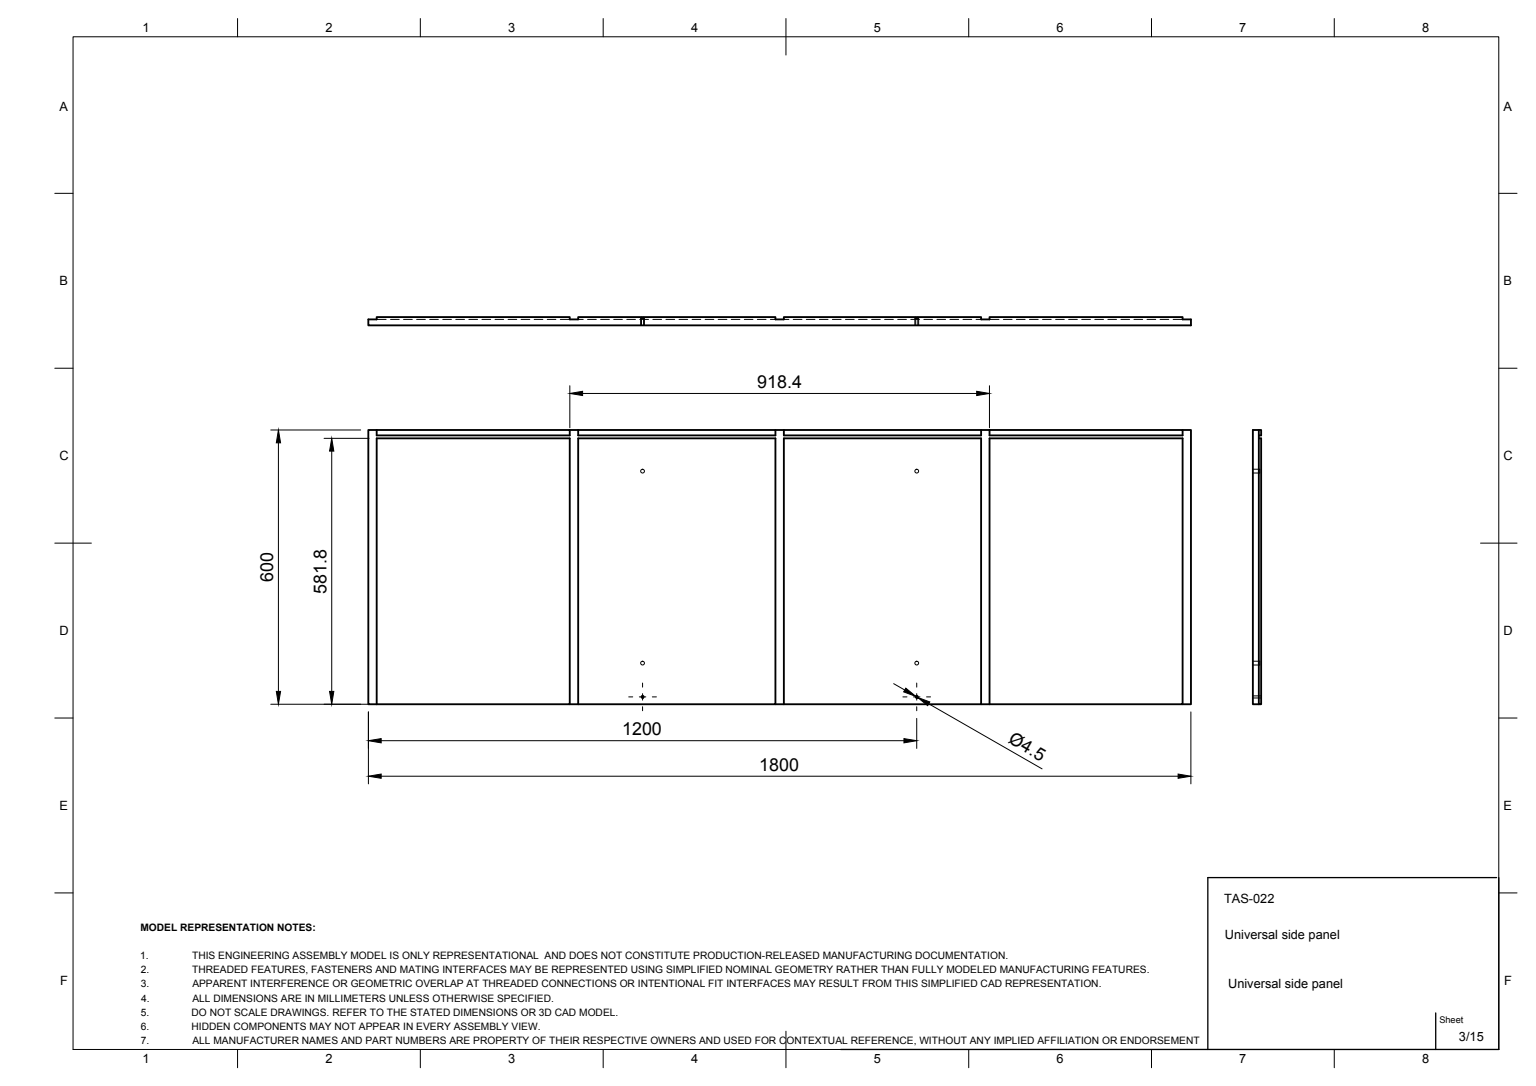
ISO-10303-21;
HEADER;
/* Generated by software containing ST-Developer
 * from STEP Tools, Inc. (www.steptools.com) 
 */

FILE_DESCRIPTION(
/* description */ (''),
/* implementation_level */ '2;1');

FILE_NAME(
/* name */ 'Universal side panel.step',
/* time_stamp */ '2026-11-15T21:02:08-08:00',
/* author */ (''),
/* organization */ (''),
/* preprocessor_version */ 'ST-DEVELOPER v20.2',
/* originating_system */ 'Autodesk Translation Framework v15.17.0.0',
/* authorisation */ '');

FILE_SCHEMA (('AUTOMOTIVE_DESIGN { 1 0 10303 214 3 1 1 }'));
ENDSEC;

DATA;
#10=MECHANICAL_DESIGN_GEOMETRIC_PRESENTATION_REPRESENTATION('',(#608),#31566);
#401=FACE_BOUND('',#1014,.T.);
#402=FACE_BOUND('',#1021,.T.);
#403=FACE_BOUND('',#1035,.T.);
#404=FACE_BOUND('',#1036,.T.);
#405=FACE_BOUND('',#1037,.T.);
#406=FACE_BOUND('',#1038,.T.);
#407=FACE_BOUND('',#1039,.T.);
#408=FACE_BOUND('',#1040,.T.);
#457=CIRCLE('',#6010,0.409999999999997);
#458=CIRCLE('',#6011,0.409999999999997);
#459=CIRCLE('',#6014,0.409999999999997);
#460=CIRCLE('',#6015,0.409999999999997);
#461=CIRCLE('',#6018,0.409999999999997);
#462=CIRCLE('',#6019,0.409999999999997);
#463=CIRCLE('',#6022,0.409999999999997);
#464=CIRCLE('',#6023,0.409999999999997);
#465=CIRCLE('',#6026,0.225000000000001);
#466=CIRCLE('',#6027,0.225000000000001);
#467=CIRCLE('',#6029,0.224999999999994);
#468=CIRCLE('',#6030,0.224999999999994);
#510=CYLINDRICAL_SURFACE('',#6009,0.409999999999997);
#511=CYLINDRICAL_SURFACE('',#6013,0.409999999999997);
#512=CYLINDRICAL_SURFACE('',#6017,0.409999999999997);
#513=CYLINDRICAL_SURFACE('',#6021,0.409999999999997);
#514=CYLINDRICAL_SURFACE('',#6025,0.225000000000001);
#515=CYLINDRICAL_SURFACE('',#6028,0.224999999999994);
#578=SHAPE_REPRESENTATION_RELATIONSHIP('SRR','None',#31642,#593);
#593=ADVANCED_BREP_SHAPE_REPRESENTATION('',(#623),#31557);
#608=STYLED_ITEM('',(#31723),#623);
#623=MANIFOLD_SOLID_BREP('Body1',#5721);
#697=FACE_OUTER_BOUND('',#986,.T.);
#698=FACE_OUTER_BOUND('',#987,.T.);
#699=FACE_OUTER_BOUND('',#988,.T.);
#700=FACE_OUTER_BOUND('',#989,.T.);
#701=FACE_OUTER_BOUND('',#990,.T.);
#702=FACE_OUTER_BOUND('',#991,.T.);
#703=FACE_OUTER_BOUND('',#992,.T.);
#704=FACE_OUTER_BOUND('',#993,.T.);
#705=FACE_OUTER_BOUND('',#994,.T.);
#706=FACE_OUTER_BOUND('',#995,.T.);
#707=FACE_OUTER_BOUND('',#996,.T.);
#708=FACE_OUTER_BOUND('',#997,.T.);
#709=FACE_OUTER_BOUND('',#998,.T.);
#710=FACE_OUTER_BOUND('',#999,.T.);
#711=FACE_OUTER_BOUND('',#1000,.T.);
#712=FACE_OUTER_BOUND('',#1001,.T.);
#713=FACE_OUTER_BOUND('',#1002,.T.);
#714=FACE_OUTER_BOUND('',#1003,.T.);
#715=FACE_OUTER_BOUND('',#1004,.T.);
#716=FACE_OUTER_BOUND('',#1005,.T.);
#717=FACE_OUTER_BOUND('',#1006,.T.);
#718=FACE_OUTER_BOUND('',#1007,.T.);
#719=FACE_OUTER_BOUND('',#1008,.T.);
#720=FACE_OUTER_BOUND('',#1009,.T.);
#721=FACE_OUTER_BOUND('',#1010,.T.);
#722=FACE_OUTER_BOUND('',#1011,.T.);
#723=FACE_OUTER_BOUND('',#1012,.T.);
#724=FACE_OUTER_BOUND('',#1013,.T.);
#725=FACE_OUTER_BOUND('',#1015,.T.);
#726=FACE_OUTER_BOUND('',#1016,.T.);
#727=FACE_OUTER_BOUND('',#1017,.T.);
#728=FACE_OUTER_BOUND('',#1018,.T.);
#729=FACE_OUTER_BOUND('',#1019,.T.);
#730=FACE_OUTER_BOUND('',#1020,.T.);
#731=FACE_OUTER_BOUND('',#1022,.T.);
#732=FACE_OUTER_BOUND('',#1023,.T.);
#733=FACE_OUTER_BOUND('',#1024,.T.);
#734=FACE_OUTER_BOUND('',#1025,.T.);
#735=FACE_OUTER_BOUND('',#1026,.T.);
#736=FACE_OUTER_BOUND('',#1027,.T.);
#737=FACE_OUTER_BOUND('',#1028,.T.);
#738=FACE_OUTER_BOUND('',#1029,.T.);
#739=FACE_OUTER_BOUND('',#1030,.T.);
#740=FACE_OUTER_BOUND('',#1031,.T.);
#741=FACE_OUTER_BOUND('',#1032,.T.);
#742=FACE_OUTER_BOUND('',#1033,.T.);
#743=FACE_OUTER_BOUND('',#1034,.T.);
#744=FACE_OUTER_BOUND('',#1041,.T.);
#986=EDGE_LOOP('',(#3945,#3946,#3947,#3948));
#987=EDGE_LOOP('',(#3949));
#988=EDGE_LOOP('',(#3950,#3951,#3952,#3953));
#989=EDGE_LOOP('',(#3954));
#990=EDGE_LOOP('',(#3955,#3956,#3957,#3958));
#991=EDGE_LOOP('',(#3959));
#992=EDGE_LOOP('',(#3960,#3961,#3962,#3963));
#993=EDGE_LOOP('',(#3964));
#994=EDGE_LOOP('',(#3965,#3966,#3967,#3968));
#995=EDGE_LOOP('',(#3969,#3970,#3971,#3972));
#996=EDGE_LOOP('',(#3973,#3974,#3975,#3976));
#997=EDGE_LOOP('',(#3977,#3978,#3979,#3980));
#998=EDGE_LOOP('',(#3981,#3982,#3983,#3984));
#999=EDGE_LOOP('',(#3985,#3986,#3987,#3988));
#1000=EDGE_LOOP('',(#3989,#3990,#3991,#3992));
#1001=EDGE_LOOP('',(#3993,#3994,#3995,#3996));
#1002=EDGE_LOOP('',(#3997,#3998,#3999,#4000));
#1003=EDGE_LOOP('',(#4001,#4002,#4003,#4004));
#1004=EDGE_LOOP('',(#4005,#4006,#4007,#4008,#4009,#4010,#4011,#4012,#4013,
#4014,#4015,#4016,#4017,#4018,#4019,#4020,#4021,#4022,#4023,#4024,#4025,
#4026,#4027,#4028,#4029,#4030,#4031,#4032,#4033,#4034,#4035,#4036,#4037,
#4038,#4039,#4040));
#1005=EDGE_LOOP('',(#4041,#4042,#4043,#4044));
#1006=EDGE_LOOP('',(#4045,#4046,#4047,#4048));
#1007=EDGE_LOOP('',(#4049,#4050,#4051,#4052));
#1008=EDGE_LOOP('',(#4053,#4054,#4055,#4056));
#1009=EDGE_LOOP('',(#4057,#4058,#4059,#4060));
#1010=EDGE_LOOP('',(#4061,#4062,#4063,#4064));
#1011=EDGE_LOOP('',(#4065,#4066,#4067,#4068));
#1012=EDGE_LOOP('',(#4069,#4070,#4071,#4072));
#1013=EDGE_LOOP('',(#4073,#4074,#4075,#4076));
#1014=EDGE_LOOP('',(#4077));
#1015=EDGE_LOOP('',(#4078,#4079,#4080,#4081));
#1016=EDGE_LOOP('',(#4082,#4083,#4084,#4085));
#1017=EDGE_LOOP('',(#4086,#4087,#4088,#4089));
#1018=EDGE_LOOP('',(#4090,#4091,#4092,#4093));
#1019=EDGE_LOOP('',(#4094,#4095,#4096,#4097));
#1020=EDGE_LOOP('',(#4098,#4099,#4100,#4101));
#1021=EDGE_LOOP('',(#4102));
#1022=EDGE_LOOP('',(#4103,#4104,#4105,#4106));
#1023=EDGE_LOOP('',(#4107,#4108,#4109,#4110));
#1024=EDGE_LOOP('',(#4111,#4112,#4113,#4114));
#1025=EDGE_LOOP('',(#4115,#4116,#4117,#4118));
#1026=EDGE_LOOP('',(#4119,#4120,#4121,#4122));
#1027=EDGE_LOOP('',(#4123,#4124,#4125,#4126));
#1028=EDGE_LOOP('',(#4127,#4128,#4129,#4130));
#1029=EDGE_LOOP('',(#4131,#4132,#4133,#4134));
#1030=EDGE_LOOP('',(#4135,#4136,#4137,#4138));
#1031=EDGE_LOOP('',(#4139,#4140,#4141,#4142,#4143,#4144,#4145,#4146,#4147,
#4148,#4149,#4150,#4151,#4152,#4153,#4154,#4155,#4156,#4157,#4158));
#1032=EDGE_LOOP('',(#4159,#4160,#4161,#4162));
#1033=EDGE_LOOP('',(#4163,#4164,#4165,#4166,#4167,#4168,#4169,#4170,#4171,
#4172,#4173,#4174,#4175,#4176,#4177,#4178,#4179,#4180,#4181,#4182));
#1034=EDGE_LOOP('',(#4183,#4184,#4185,#4186));
#1035=EDGE_LOOP('',(#4187));
#1036=EDGE_LOOP('',(#4188));
#1037=EDGE_LOOP('',(#4189));
#1038=EDGE_LOOP('',(#4190));
#1039=EDGE_LOOP('',(#4191));
#1040=EDGE_LOOP('',(#4192));
#1041=EDGE_LOOP('',(#4193,#4194,#4195,#4196));
#1325=LINE('',#7903,#1832);
#1326=LINE('',#7910,#1833);
#1327=LINE('',#7917,#1834);
#1328=LINE('',#7924,#1835);
#1329=LINE('',#7931,#1836);
#1330=LINE('',#7937,#1837);
#1331=LINE('',#7942,#1838);
#1332=LINE('',#7944,#1839);
#1333=LINE('',#7946,#1840);
#1334=LINE('',#7947,#1841);
#1335=LINE('',#7951,#1842);
#1336=LINE('',#7953,#1843);
#1337=LINE('',#7955,#1844);
#1338=LINE('',#7956,#1845);
#1339=LINE('',#7960,#1846);
#1340=LINE('',#7962,#1847);
#1341=LINE('',#7964,#1848);
#1342=LINE('',#7965,#1849);
#1343=LINE('',#7969,#1850);
#1344=LINE('',#7971,#1851);
#1345=LINE('',#7973,#1852);
#1346=LINE('',#7974,#1853);
#1347=LINE('',#7978,#1854);
#1348=LINE('',#7980,#1855);
#1349=LINE('',#7982,#1856);
#1350=LINE('',#7983,#1857);
#1351=LINE('',#7987,#1858);
#1352=LINE('',#7989,#1859);
#1353=LINE('',#7991,#1860);
#1354=LINE('',#7992,#1861);
#1355=LINE('',#7996,#1862);
#1356=LINE('',#7998,#1863);
#1357=LINE('',#8000,#1864);
#1358=LINE('',#8001,#1865);
#1359=LINE('',#8005,#1866);
#1360=LINE('',#8007,#1867);
#1361=LINE('',#8009,#1868);
#1362=LINE('',#8010,#1869);
#1363=LINE('',#8013,#1870);
#1364=LINE('',#8015,#1871);
#1365=LINE('',#8017,#1872);
#1366=LINE('',#8019,#1873);
#1367=LINE('',#8020,#1874);
#1368=LINE('',#8022,#1875);
#1369=LINE('',#8024,#1876);
#1370=LINE('',#8025,#1877);
#1371=LINE('',#8027,#1878);
#1372=LINE('',#8029,#1879);
#1373=LINE('',#8030,#1880);
#1374=LINE('',#8032,#1881);
#1375=LINE('',#8034,#1882);
#1376=LINE('',#8035,#1883);
#1377=LINE('',#8037,#1884);
#1378=LINE('',#8039,#1885);
#1379=LINE('',#8041,#1886);
#1380=LINE('',#8043,#1887);
#1381=LINE('',#8044,#1888);
#1382=LINE('',#8046,#1889);
#1383=LINE('',#8048,#1890);
#1384=LINE('',#8049,#1891);
#1385=LINE('',#8051,#1892);
#1386=LINE('',#8053,#1893);
#1387=LINE('',#8054,#1894);
#1388=LINE('',#8056,#1895);
#1389=LINE('',#8058,#1896);
#1390=LINE('',#8059,#1897);
#1391=LINE('',#8062,#1898);
#1392=LINE('',#8063,#1899);
#1393=LINE('',#8066,#1900);
#1394=LINE('',#8067,#1901);
#1395=LINE('',#8070,#1902);
#1396=LINE('',#8071,#1903);
#1397=LINE('',#8074,#1904);
#1398=LINE('',#8075,#1905);
#1399=LINE('',#8077,#1906);
#1400=LINE('',#8079,#1907);
#1401=LINE('',#8082,#1908);
#1402=LINE('',#8083,#1909);
#1403=LINE('',#8086,#1910);
#1404=LINE('',#8087,#1911);
#1405=LINE('',#8090,#1912);
#1406=LINE('',#8091,#1913);
#1407=LINE('',#8094,#1914);
#1408=LINE('',#8095,#1915);
#1409=LINE('',#8097,#1916);
#1410=LINE('',#8099,#1917);
#1411=LINE('',#8102,#1918);
#1412=LINE('',#8103,#1919);
#1413=LINE('',#8106,#1920);
#1414=LINE('',#8107,#1921);
#1415=LINE('',#8110,#1922);
#1416=LINE('',#8111,#1923);
#1417=LINE('',#8114,#1924);
#1418=LINE('',#8115,#1925);
#1419=LINE('',#8117,#1926);
#1420=LINE('',#8119,#1927);
#1421=LINE('',#8122,#1928);
#1422=LINE('',#8123,#1929);
#1423=LINE('',#8126,#1930);
#1424=LINE('',#8127,#1931);
#1425=LINE('',#8130,#1932);
#1426=LINE('',#8131,#1933);
#1427=LINE('',#8134,#1934);
#1428=LINE('',#8135,#1935);
#1429=LINE('',#8137,#1936);
#1430=LINE('',#8139,#1937);
#1431=LINE('',#8142,#1938);
#1432=LINE('',#8144,#1939);
#1433=LINE('',#8145,#1940);
#1434=LINE('',#8148,#1941);
#1435=LINE('',#8149,#1942);
#1436=LINE('',#8152,#1943);
#1437=LINE('',#8153,#1944);
#1438=LINE('',#8155,#1945);
#1832=VECTOR('',#6631,0.409999999999997);
#1833=VECTOR('',#6640,0.409999999999997);
#1834=VECTOR('',#6649,0.409999999999997);
#1835=VECTOR('',#6658,0.409999999999997);
#1836=VECTOR('',#6667,0.225000000000001);
#1837=VECTOR('',#6674,0.224999999999994);
#1838=VECTOR('',#6679,1.);
#1839=VECTOR('',#6680,1.);
#1840=VECTOR('',#6681,1.);
#1841=VECTOR('',#6682,1.);
#1842=VECTOR('',#6685,1.);
#1843=VECTOR('',#6686,1.);
#1844=VECTOR('',#6687,1.);
#1845=VECTOR('',#6688,1.);
#1846=VECTOR('',#6691,1.);
#1847=VECTOR('',#6692,1.);
#1848=VECTOR('',#6693,1.);
#1849=VECTOR('',#6694,1.);
#1850=VECTOR('',#6697,1.);
#1851=VECTOR('',#6698,1.);
#1852=VECTOR('',#6699,1.);
#1853=VECTOR('',#6700,1.);
#1854=VECTOR('',#6703,1.);
#1855=VECTOR('',#6704,1.);
#1856=VECTOR('',#6705,1.);
#1857=VECTOR('',#6706,1.);
#1858=VECTOR('',#6709,1.);
#1859=VECTOR('',#6710,1.);
#1860=VECTOR('',#6711,1.);
#1861=VECTOR('',#6712,1.);
#1862=VECTOR('',#6715,1.);
#1863=VECTOR('',#6716,1.);
#1864=VECTOR('',#6717,1.);
#1865=VECTOR('',#6718,1.);
#1866=VECTOR('',#6721,1.);
#1867=VECTOR('',#6722,1.);
#1868=VECTOR('',#6723,1.);
#1869=VECTOR('',#6724,1.);
#1870=VECTOR('',#6727,1.);
#1871=VECTOR('',#6728,1.);
#1872=VECTOR('',#6729,1.);
#1873=VECTOR('',#6730,1.);
#1874=VECTOR('',#6731,1.);
#1875=VECTOR('',#6732,1.);
#1876=VECTOR('',#6733,1.);
#1877=VECTOR('',#6734,1.);
#1878=VECTOR('',#6735,1.);
#1879=VECTOR('',#6736,1.);
#1880=VECTOR('',#6737,1.);
#1881=VECTOR('',#6738,1.);
#1882=VECTOR('',#6739,1.);
#1883=VECTOR('',#6740,1.);
#1884=VECTOR('',#6741,1.);
#1885=VECTOR('',#6742,1.);
#1886=VECTOR('',#6743,1.);
#1887=VECTOR('',#6744,1.);
#1888=VECTOR('',#6745,1.);
#1889=VECTOR('',#6746,1.);
#1890=VECTOR('',#6747,1.);
#1891=VECTOR('',#6748,1.);
#1892=VECTOR('',#6749,1.);
#1893=VECTOR('',#6750,1.);
#1894=VECTOR('',#6751,1.);
#1895=VECTOR('',#6752,1.);
#1896=VECTOR('',#6753,1.);
#1897=VECTOR('',#6754,1.);
#1898=VECTOR('',#6757,1.);
#1899=VECTOR('',#6758,1.);
#1900=VECTOR('',#6761,1.);
#1901=VECTOR('',#6762,1.);
#1902=VECTOR('',#6765,1.);
#1903=VECTOR('',#6766,1.);
#1904=VECTOR('',#6769,1.);
#1905=VECTOR('',#6770,1.);
#1906=VECTOR('',#6773,1.);
#1907=VECTOR('',#6776,1.);
#1908=VECTOR('',#6779,1.);
#1909=VECTOR('',#6780,1.);
#1910=VECTOR('',#6783,1.);
#1911=VECTOR('',#6784,1.);
#1912=VECTOR('',#6787,1.);
#1913=VECTOR('',#6788,1.);
#1914=VECTOR('',#6791,1.);
#1915=VECTOR('',#6792,1.);
#1916=VECTOR('',#6795,1.);
#1917=VECTOR('',#6798,1.);
#1918=VECTOR('',#6801,1.);
#1919=VECTOR('',#6802,1.);
#1920=VECTOR('',#6805,1.);
#1921=VECTOR('',#6806,1.);
#1922=VECTOR('',#6809,1.);
#1923=VECTOR('',#6810,1.);
#1924=VECTOR('',#6813,1.);
#1925=VECTOR('',#6814,1.);
#1926=VECTOR('',#6817,1.);
#1927=VECTOR('',#6820,1.);
#1928=VECTOR('',#6823,1.);
#1929=VECTOR('',#6824,1.);
#1930=VECTOR('',#6827,1.);
#1931=VECTOR('',#6828,1.);
#1932=VECTOR('',#6831,1.);
#1933=VECTOR('',#6832,1.);
#1934=VECTOR('',#6835,1.);
#1935=VECTOR('',#6836,1.);
#1936=VECTOR('',#6839,1.);
#1937=VECTOR('',#6842,1.);
#1938=VECTOR('',#6845,1.);
#1939=VECTOR('',#6846,1.);
#1940=VECTOR('',#6847,1.);
#1941=VECTOR('',#6850,1.);
#1942=VECTOR('',#6851,1.);
#1943=VECTOR('',#6854,1.);
#1944=VECTOR('',#6855,1.);
#1945=VECTOR('',#6858,1.);
#2326=VERTEX_POINT('',#7900);
#2327=VERTEX_POINT('',#7902);
#2328=VERTEX_POINT('',#7907);
#2329=VERTEX_POINT('',#7909);
#2330=VERTEX_POINT('',#7914);
#2331=VERTEX_POINT('',#7916);
#2332=VERTEX_POINT('',#7921);
#2333=VERTEX_POINT('',#7923);
#2334=VERTEX_POINT('',#7928);
#2335=VERTEX_POINT('',#7930);
#2336=VERTEX_POINT('',#7934);
#2337=VERTEX_POINT('',#7936);
#2338=VERTEX_POINT('',#7940);
#2339=VERTEX_POINT('',#7941);
#2340=VERTEX_POINT('',#7943);
#2341=VERTEX_POINT('',#7945);
#2342=VERTEX_POINT('',#7949);
#2343=VERTEX_POINT('',#7950);
#2344=VERTEX_POINT('',#7952);
#2345=VERTEX_POINT('',#7954);
#2346=VERTEX_POINT('',#7958);
#2347=VERTEX_POINT('',#7959);
#2348=VERTEX_POINT('',#7961);
#2349=VERTEX_POINT('',#7963);
#2350=VERTEX_POINT('',#7967);
#2351=VERTEX_POINT('',#7968);
#2352=VERTEX_POINT('',#7970);
#2353=VERTEX_POINT('',#7972);
#2354=VERTEX_POINT('',#7976);
#2355=VERTEX_POINT('',#7977);
#2356=VERTEX_POINT('',#7979);
#2357=VERTEX_POINT('',#7981);
#2358=VERTEX_POINT('',#7985);
#2359=VERTEX_POINT('',#7986);
#2360=VERTEX_POINT('',#7988);
#2361=VERTEX_POINT('',#7990);
#2362=VERTEX_POINT('',#7994);
#2363=VERTEX_POINT('',#7995);
#2364=VERTEX_POINT('',#7997);
#2365=VERTEX_POINT('',#7999);
#2366=VERTEX_POINT('',#8003);
#2367=VERTEX_POINT('',#8004);
#2368=VERTEX_POINT('',#8006);
#2369=VERTEX_POINT('',#8008);
#2370=VERTEX_POINT('',#8012);
#2371=VERTEX_POINT('',#8014);
#2372=VERTEX_POINT('',#8016);
#2373=VERTEX_POINT('',#8018);
#2374=VERTEX_POINT('',#8021);
#2375=VERTEX_POINT('',#8023);
#2376=VERTEX_POINT('',#8026);
#2377=VERTEX_POINT('',#8028);
#2378=VERTEX_POINT('',#8031);
#2379=VERTEX_POINT('',#8033);
#2380=VERTEX_POINT('',#8036);
#2381=VERTEX_POINT('',#8038);
#2382=VERTEX_POINT('',#8040);
#2383=VERTEX_POINT('',#8042);
#2384=VERTEX_POINT('',#8045);
#2385=VERTEX_POINT('',#8047);
#2386=VERTEX_POINT('',#8050);
#2387=VERTEX_POINT('',#8052);
#2388=VERTEX_POINT('',#8055);
#2389=VERTEX_POINT('',#8057);
#2390=VERTEX_POINT('',#8061);
#2391=VERTEX_POINT('',#8065);
#2392=VERTEX_POINT('',#8069);
#2393=VERTEX_POINT('',#8073);
#2394=VERTEX_POINT('',#8081);
#2395=VERTEX_POINT('',#8085);
#2396=VERTEX_POINT('',#8089);
#2397=VERTEX_POINT('',#8093);
#2398=VERTEX_POINT('',#8101);
#2399=VERTEX_POINT('',#8105);
#2400=VERTEX_POINT('',#8109);
#2401=VERTEX_POINT('',#8113);
#2402=VERTEX_POINT('',#8121);
#2403=VERTEX_POINT('',#8125);
#2404=VERTEX_POINT('',#8129);
#2405=VERTEX_POINT('',#8133);
#2406=VERTEX_POINT('',#8141);
#2407=VERTEX_POINT('',#8143);
#2408=VERTEX_POINT('',#8147);
#2409=VERTEX_POINT('',#8151);
#2968=EDGE_CURVE('',#2326,#2326,#457,.T.);
#2969=EDGE_CURVE('',#2326,#2327,#1325,.T.);
#2970=EDGE_CURVE('',#2327,#2327,#458,.T.);
#2971=EDGE_CURVE('',#2328,#2328,#459,.T.);
#2972=EDGE_CURVE('',#2328,#2329,#1326,.T.);
#2973=EDGE_CURVE('',#2329,#2329,#460,.T.);
#2974=EDGE_CURVE('',#2330,#2330,#461,.T.);
#2975=EDGE_CURVE('',#2330,#2331,#1327,.T.);
#2976=EDGE_CURVE('',#2331,#2331,#462,.T.);
#2977=EDGE_CURVE('',#2332,#2332,#463,.T.);
#2978=EDGE_CURVE('',#2332,#2333,#1328,.T.);
#2979=EDGE_CURVE('',#2333,#2333,#464,.T.);
#2980=EDGE_CURVE('',#2334,#2334,#465,.T.);
#2981=EDGE_CURVE('',#2334,#2335,#1329,.T.);
#2982=EDGE_CURVE('',#2335,#2335,#466,.T.);
#2983=EDGE_CURVE('',#2336,#2336,#467,.T.);
#2984=EDGE_CURVE('',#2336,#2337,#1330,.T.);
#2985=EDGE_CURVE('',#2337,#2337,#468,.T.);
#2986=EDGE_CURVE('',#2338,#2339,#1331,.T.);
#2987=EDGE_CURVE('',#2340,#2338,#1332,.T.);
#2988=EDGE_CURVE('',#2341,#2340,#1333,.T.);
#2989=EDGE_CURVE('',#2339,#2341,#1334,.T.);
#2990=EDGE_CURVE('',#2342,#2343,#1335,.T.);
#2991=EDGE_CURVE('',#2344,#2342,#1336,.T.);
#2992=EDGE_CURVE('',#2345,#2344,#1337,.T.);
#2993=EDGE_CURVE('',#2343,#2345,#1338,.T.);
#2994=EDGE_CURVE('',#2346,#2347,#1339,.T.);
#2995=EDGE_CURVE('',#2348,#2346,#1340,.T.);
#2996=EDGE_CURVE('',#2349,#2348,#1341,.T.);
#2997=EDGE_CURVE('',#2347,#2349,#1342,.T.);
#2998=EDGE_CURVE('',#2350,#2351,#1343,.T.);
#2999=EDGE_CURVE('',#2352,#2350,#1344,.T.);
#3000=EDGE_CURVE('',#2353,#2352,#1345,.T.);
#3001=EDGE_CURVE('',#2351,#2353,#1346,.T.);
#3002=EDGE_CURVE('',#2354,#2355,#1347,.T.);
#3003=EDGE_CURVE('',#2356,#2354,#1348,.T.);
#3004=EDGE_CURVE('',#2357,#2356,#1349,.T.);
#3005=EDGE_CURVE('',#2357,#2355,#1350,.T.);
#3006=EDGE_CURVE('',#2358,#2359,#1351,.T.);
#3007=EDGE_CURVE('',#2360,#2358,#1352,.T.);
#3008=EDGE_CURVE('',#2361,#2360,#1353,.T.);
#3009=EDGE_CURVE('',#2361,#2359,#1354,.T.);
#3010=EDGE_CURVE('',#2362,#2363,#1355,.T.);
#3011=EDGE_CURVE('',#2364,#2362,#1356,.T.);
#3012=EDGE_CURVE('',#2365,#2364,#1357,.T.);
#3013=EDGE_CURVE('',#2365,#2363,#1358,.T.);
#3014=EDGE_CURVE('',#2366,#2367,#1359,.T.);
#3015=EDGE_CURVE('',#2368,#2366,#1360,.T.);
#3016=EDGE_CURVE('',#2369,#2368,#1361,.T.);
#3017=EDGE_CURVE('',#2369,#2367,#1362,.T.);
#3018=EDGE_CURVE('',#2370,#2350,#1363,.T.);
#3019=EDGE_CURVE('',#2371,#2370,#1364,.T.);
#3020=EDGE_CURVE('',#2372,#2371,#1365,.T.);
#3021=EDGE_CURVE('',#2373,#2372,#1366,.T.);
#3022=EDGE_CURVE('',#2367,#2373,#1367,.T.);
#3023=EDGE_CURVE('',#2369,#2374,#1368,.T.);
#3024=EDGE_CURVE('',#2375,#2374,#1369,.T.);
#3025=EDGE_CURVE('',#2363,#2375,#1370,.T.);
#3026=EDGE_CURVE('',#2365,#2376,#1371,.T.);
#3027=EDGE_CURVE('',#2377,#2376,#1372,.T.);
#3028=EDGE_CURVE('',#2359,#2377,#1373,.T.);
#3029=EDGE_CURVE('',#2361,#2378,#1374,.T.);
#3030=EDGE_CURVE('',#2379,#2378,#1375,.T.);
#3031=EDGE_CURVE('',#2355,#2379,#1376,.T.);
#3032=EDGE_CURVE('',#2357,#2380,#1377,.T.);
#3033=EDGE_CURVE('',#2381,#2380,#1378,.T.);
#3034=EDGE_CURVE('',#2382,#2381,#1379,.T.);
#3035=EDGE_CURVE('',#2383,#2382,#1380,.T.);
#3036=EDGE_CURVE('',#2383,#2348,#1381,.T.);
#3037=EDGE_CURVE('',#2384,#2346,#1382,.T.);
#3038=EDGE_CURVE('',#2385,#2384,#1383,.T.);
#3039=EDGE_CURVE('',#2385,#2344,#1384,.T.);
#3040=EDGE_CURVE('',#2386,#2342,#1385,.T.);
#3041=EDGE_CURVE('',#2387,#2386,#1386,.T.);
#3042=EDGE_CURVE('',#2387,#2340,#1387,.T.);
#3043=EDGE_CURVE('',#2388,#2338,#1388,.T.);
#3044=EDGE_CURVE('',#2389,#2388,#1389,.T.);
#3045=EDGE_CURVE('',#2389,#2352,#1390,.T.);
#3046=EDGE_CURVE('',#2390,#2373,#1391,.T.);
#3047=EDGE_CURVE('',#2366,#2390,#1392,.T.);
#3048=EDGE_CURVE('',#2391,#2351,#1393,.T.);
#3049=EDGE_CURVE('',#2370,#2391,#1394,.T.);
#3050=EDGE_CURVE('',#2392,#2390,#1395,.T.);
#3051=EDGE_CURVE('',#2392,#2368,#1396,.T.);
#3052=EDGE_CURVE('',#2353,#2393,#1397,.T.);
#3053=EDGE_CURVE('',#2393,#2391,#1398,.T.);
#3054=EDGE_CURVE('',#2374,#2392,#1399,.T.);
#3055=EDGE_CURVE('',#2393,#2389,#1400,.T.);
#3056=EDGE_CURVE('',#2394,#2375,#1401,.T.);
#3057=EDGE_CURVE('',#2362,#2394,#1402,.T.);
#3058=EDGE_CURVE('',#2395,#2339,#1403,.T.);
#3059=EDGE_CURVE('',#2388,#2395,#1404,.T.);
#3060=EDGE_CURVE('',#2396,#2394,#1405,.T.);
#3061=EDGE_CURVE('',#2396,#2364,#1406,.T.);
#3062=EDGE_CURVE('',#2341,#2397,#1407,.T.);
#3063=EDGE_CURVE('',#2397,#2395,#1408,.T.);
#3064=EDGE_CURVE('',#2376,#2396,#1409,.T.);
#3065=EDGE_CURVE('',#2397,#2387,#1410,.T.);
#3066=EDGE_CURVE('',#2398,#2377,#1411,.T.);
#3067=EDGE_CURVE('',#2358,#2398,#1412,.T.);
#3068=EDGE_CURVE('',#2399,#2343,#1413,.T.);
#3069=EDGE_CURVE('',#2386,#2399,#1414,.T.);
#3070=EDGE_CURVE('',#2400,#2398,#1415,.T.);
#3071=EDGE_CURVE('',#2400,#2360,#1416,.T.);
#3072=EDGE_CURVE('',#2345,#2401,#1417,.T.);
#3073=EDGE_CURVE('',#2401,#2399,#1418,.T.);
#3074=EDGE_CURVE('',#2378,#2400,#1419,.T.);
#3075=EDGE_CURVE('',#2401,#2385,#1420,.T.);
#3076=EDGE_CURVE('',#2402,#2379,#1421,.T.);
#3077=EDGE_CURVE('',#2354,#2402,#1422,.T.);
#3078=EDGE_CURVE('',#2403,#2347,#1423,.T.);
#3079=EDGE_CURVE('',#2384,#2403,#1424,.T.);
#3080=EDGE_CURVE('',#2404,#2402,#1425,.T.);
#3081=EDGE_CURVE('',#2404,#2356,#1426,.T.);
#3082=EDGE_CURVE('',#2349,#2405,#1427,.T.);
#3083=EDGE_CURVE('',#2405,#2403,#1428,.T.);
#3084=EDGE_CURVE('',#2380,#2404,#1429,.T.);
#3085=EDGE_CURVE('',#2405,#2383,#1430,.T.);
#3086=EDGE_CURVE('',#2382,#2406,#1431,.T.);
#3087=EDGE_CURVE('',#2406,#2407,#1432,.T.);
#3088=EDGE_CURVE('',#2371,#2407,#1433,.T.);
#3089=EDGE_CURVE('',#2408,#2381,#1434,.T.);
#3090=EDGE_CURVE('',#2406,#2408,#1435,.T.);
#3091=EDGE_CURVE('',#2409,#2372,#1436,.T.);
#3092=EDGE_CURVE('',#2408,#2409,#1437,.T.);
#3093=EDGE_CURVE('',#2407,#2409,#1438,.T.);
#3945=ORIENTED_EDGE('',*,*,#2968,.F.);
#3946=ORIENTED_EDGE('',*,*,#2969,.T.);
#3947=ORIENTED_EDGE('',*,*,#2970,.T.);
#3948=ORIENTED_EDGE('',*,*,#2969,.F.);
#3949=ORIENTED_EDGE('',*,*,#2970,.F.);
#3950=ORIENTED_EDGE('',*,*,#2971,.F.);
#3951=ORIENTED_EDGE('',*,*,#2972,.T.);
#3952=ORIENTED_EDGE('',*,*,#2973,.T.);
#3953=ORIENTED_EDGE('',*,*,#2972,.F.);
#3954=ORIENTED_EDGE('',*,*,#2973,.F.);
#3955=ORIENTED_EDGE('',*,*,#2974,.F.);
#3956=ORIENTED_EDGE('',*,*,#2975,.T.);
#3957=ORIENTED_EDGE('',*,*,#2976,.T.);
#3958=ORIENTED_EDGE('',*,*,#2975,.F.);
#3959=ORIENTED_EDGE('',*,*,#2976,.F.);
#3960=ORIENTED_EDGE('',*,*,#2977,.F.);
#3961=ORIENTED_EDGE('',*,*,#2978,.T.);
#3962=ORIENTED_EDGE('',*,*,#2979,.T.);
#3963=ORIENTED_EDGE('',*,*,#2978,.F.);
#3964=ORIENTED_EDGE('',*,*,#2979,.F.);
#3965=ORIENTED_EDGE('',*,*,#2980,.F.);
#3966=ORIENTED_EDGE('',*,*,#2981,.T.);
#3967=ORIENTED_EDGE('',*,*,#2982,.F.);
#3968=ORIENTED_EDGE('',*,*,#2981,.F.);
#3969=ORIENTED_EDGE('',*,*,#2983,.F.);
#3970=ORIENTED_EDGE('',*,*,#2984,.T.);
#3971=ORIENTED_EDGE('',*,*,#2985,.F.);
#3972=ORIENTED_EDGE('',*,*,#2984,.F.);
#3973=ORIENTED_EDGE('',*,*,#2986,.F.);
#3974=ORIENTED_EDGE('',*,*,#2987,.F.);
#3975=ORIENTED_EDGE('',*,*,#2988,.F.);
#3976=ORIENTED_EDGE('',*,*,#2989,.F.);
#3977=ORIENTED_EDGE('',*,*,#2990,.F.);
#3978=ORIENTED_EDGE('',*,*,#2991,.F.);
#3979=ORIENTED_EDGE('',*,*,#2992,.F.);
#3980=ORIENTED_EDGE('',*,*,#2993,.F.);
#3981=ORIENTED_EDGE('',*,*,#2994,.F.);
#3982=ORIENTED_EDGE('',*,*,#2995,.F.);
#3983=ORIENTED_EDGE('',*,*,#2996,.F.);
#3984=ORIENTED_EDGE('',*,*,#2997,.F.);
#3985=ORIENTED_EDGE('',*,*,#2998,.F.);
#3986=ORIENTED_EDGE('',*,*,#2999,.F.);
#3987=ORIENTED_EDGE('',*,*,#3000,.F.);
#3988=ORIENTED_EDGE('',*,*,#3001,.F.);
#3989=ORIENTED_EDGE('',*,*,#3002,.F.);
#3990=ORIENTED_EDGE('',*,*,#3003,.F.);
#3991=ORIENTED_EDGE('',*,*,#3004,.F.);
#3992=ORIENTED_EDGE('',*,*,#3005,.T.);
#3993=ORIENTED_EDGE('',*,*,#3006,.F.);
#3994=ORIENTED_EDGE('',*,*,#3007,.F.);
#3995=ORIENTED_EDGE('',*,*,#3008,.F.);
#3996=ORIENTED_EDGE('',*,*,#3009,.T.);
#3997=ORIENTED_EDGE('',*,*,#3010,.F.);
#3998=ORIENTED_EDGE('',*,*,#3011,.F.);
#3999=ORIENTED_EDGE('',*,*,#3012,.F.);
#4000=ORIENTED_EDGE('',*,*,#3013,.T.);
#4001=ORIENTED_EDGE('',*,*,#3014,.F.);
#4002=ORIENTED_EDGE('',*,*,#3015,.F.);
#4003=ORIENTED_EDGE('',*,*,#3016,.F.);
#4004=ORIENTED_EDGE('',*,*,#3017,.T.);
#4005=ORIENTED_EDGE('',*,*,#3018,.F.);
#4006=ORIENTED_EDGE('',*,*,#3019,.F.);
#4007=ORIENTED_EDGE('',*,*,#3020,.F.);
#4008=ORIENTED_EDGE('',*,*,#3021,.F.);
#4009=ORIENTED_EDGE('',*,*,#3022,.F.);
#4010=ORIENTED_EDGE('',*,*,#3017,.F.);
#4011=ORIENTED_EDGE('',*,*,#3023,.T.);
#4012=ORIENTED_EDGE('',*,*,#3024,.F.);
#4013=ORIENTED_EDGE('',*,*,#3025,.F.);
#4014=ORIENTED_EDGE('',*,*,#3013,.F.);
#4015=ORIENTED_EDGE('',*,*,#3026,.T.);
#4016=ORIENTED_EDGE('',*,*,#3027,.F.);
#4017=ORIENTED_EDGE('',*,*,#3028,.F.);
#4018=ORIENTED_EDGE('',*,*,#3009,.F.);
#4019=ORIENTED_EDGE('',*,*,#3029,.T.);
#4020=ORIENTED_EDGE('',*,*,#3030,.F.);
#4021=ORIENTED_EDGE('',*,*,#3031,.F.);
#4022=ORIENTED_EDGE('',*,*,#3005,.F.);
#4023=ORIENTED_EDGE('',*,*,#3032,.T.);
#4024=ORIENTED_EDGE('',*,*,#3033,.F.);
#4025=ORIENTED_EDGE('',*,*,#3034,.F.);
#4026=ORIENTED_EDGE('',*,*,#3035,.F.);
#4027=ORIENTED_EDGE('',*,*,#3036,.T.);
#4028=ORIENTED_EDGE('',*,*,#2995,.T.);
#4029=ORIENTED_EDGE('',*,*,#3037,.F.);
#4030=ORIENTED_EDGE('',*,*,#3038,.F.);
#4031=ORIENTED_EDGE('',*,*,#3039,.T.);
#4032=ORIENTED_EDGE('',*,*,#2991,.T.);
#4033=ORIENTED_EDGE('',*,*,#3040,.F.);
#4034=ORIENTED_EDGE('',*,*,#3041,.F.);
#4035=ORIENTED_EDGE('',*,*,#3042,.T.);
#4036=ORIENTED_EDGE('',*,*,#2987,.T.);
#4037=ORIENTED_EDGE('',*,*,#3043,.F.);
#4038=ORIENTED_EDGE('',*,*,#3044,.F.);
#4039=ORIENTED_EDGE('',*,*,#3045,.T.);
#4040=ORIENTED_EDGE('',*,*,#2999,.T.);
#4041=ORIENTED_EDGE('',*,*,#3014,.T.);
#4042=ORIENTED_EDGE('',*,*,#3022,.T.);
#4043=ORIENTED_EDGE('',*,*,#3046,.F.);
#4044=ORIENTED_EDGE('',*,*,#3047,.F.);
#4045=ORIENTED_EDGE('',*,*,#2998,.T.);
#4046=ORIENTED_EDGE('',*,*,#3048,.F.);
#4047=ORIENTED_EDGE('',*,*,#3049,.F.);
#4048=ORIENTED_EDGE('',*,*,#3018,.T.);
#4049=ORIENTED_EDGE('',*,*,#3015,.T.);
#4050=ORIENTED_EDGE('',*,*,#3047,.T.);
#4051=ORIENTED_EDGE('',*,*,#3050,.F.);
#4052=ORIENTED_EDGE('',*,*,#3051,.T.);
#4053=ORIENTED_EDGE('',*,*,#3001,.T.);
#4054=ORIENTED_EDGE('',*,*,#3052,.T.);
#4055=ORIENTED_EDGE('',*,*,#3053,.T.);
#4056=ORIENTED_EDGE('',*,*,#3048,.T.);
#4057=ORIENTED_EDGE('',*,*,#3016,.T.);
#4058=ORIENTED_EDGE('',*,*,#3051,.F.);
#4059=ORIENTED_EDGE('',*,*,#3054,.F.);
#4060=ORIENTED_EDGE('',*,*,#3023,.F.);
#4061=ORIENTED_EDGE('',*,*,#3000,.T.);
#4062=ORIENTED_EDGE('',*,*,#3045,.F.);
#4063=ORIENTED_EDGE('',*,*,#3055,.F.);
#4064=ORIENTED_EDGE('',*,*,#3052,.F.);
#4065=ORIENTED_EDGE('',*,*,#3010,.T.);
#4066=ORIENTED_EDGE('',*,*,#3025,.T.);
#4067=ORIENTED_EDGE('',*,*,#3056,.F.);
#4068=ORIENTED_EDGE('',*,*,#3057,.F.);
#4069=ORIENTED_EDGE('',*,*,#2986,.T.);
#4070=ORIENTED_EDGE('',*,*,#3058,.F.);
#4071=ORIENTED_EDGE('',*,*,#3059,.F.);
#4072=ORIENTED_EDGE('',*,*,#3043,.T.);
#4073=ORIENTED_EDGE('',*,*,#3011,.T.);
#4074=ORIENTED_EDGE('',*,*,#3057,.T.);
#4075=ORIENTED_EDGE('',*,*,#3060,.F.);
#4076=ORIENTED_EDGE('',*,*,#3061,.T.);
#4077=ORIENTED_EDGE('',*,*,#2983,.T.);
#4078=ORIENTED_EDGE('',*,*,#2989,.T.);
#4079=ORIENTED_EDGE('',*,*,#3062,.T.);
#4080=ORIENTED_EDGE('',*,*,#3063,.T.);
#4081=ORIENTED_EDGE('',*,*,#3058,.T.);
#4082=ORIENTED_EDGE('',*,*,#3012,.T.);
#4083=ORIENTED_EDGE('',*,*,#3061,.F.);
#4084=ORIENTED_EDGE('',*,*,#3064,.F.);
#4085=ORIENTED_EDGE('',*,*,#3026,.F.);
#4086=ORIENTED_EDGE('',*,*,#2988,.T.);
#4087=ORIENTED_EDGE('',*,*,#3042,.F.);
#4088=ORIENTED_EDGE('',*,*,#3065,.F.);
#4089=ORIENTED_EDGE('',*,*,#3062,.F.);
#4090=ORIENTED_EDGE('',*,*,#3006,.T.);
#4091=ORIENTED_EDGE('',*,*,#3028,.T.);
#4092=ORIENTED_EDGE('',*,*,#3066,.F.);
#4093=ORIENTED_EDGE('',*,*,#3067,.F.);
#4094=ORIENTED_EDGE('',*,*,#2990,.T.);
#4095=ORIENTED_EDGE('',*,*,#3068,.F.);
#4096=ORIENTED_EDGE('',*,*,#3069,.F.);
#4097=ORIENTED_EDGE('',*,*,#3040,.T.);
#4098=ORIENTED_EDGE('',*,*,#3007,.T.);
#4099=ORIENTED_EDGE('',*,*,#3067,.T.);
#4100=ORIENTED_EDGE('',*,*,#3070,.F.);
#4101=ORIENTED_EDGE('',*,*,#3071,.T.);
#4102=ORIENTED_EDGE('',*,*,#2980,.T.);
#4103=ORIENTED_EDGE('',*,*,#2993,.T.);
#4104=ORIENTED_EDGE('',*,*,#3072,.T.);
#4105=ORIENTED_EDGE('',*,*,#3073,.T.);
#4106=ORIENTED_EDGE('',*,*,#3068,.T.);
#4107=ORIENTED_EDGE('',*,*,#3008,.T.);
#4108=ORIENTED_EDGE('',*,*,#3071,.F.);
#4109=ORIENTED_EDGE('',*,*,#3074,.F.);
#4110=ORIENTED_EDGE('',*,*,#3029,.F.);
#4111=ORIENTED_EDGE('',*,*,#2992,.T.);
#4112=ORIENTED_EDGE('',*,*,#3039,.F.);
#4113=ORIENTED_EDGE('',*,*,#3075,.F.);
#4114=ORIENTED_EDGE('',*,*,#3072,.F.);
#4115=ORIENTED_EDGE('',*,*,#3002,.T.);
#4116=ORIENTED_EDGE('',*,*,#3031,.T.);
#4117=ORIENTED_EDGE('',*,*,#3076,.F.);
#4118=ORIENTED_EDGE('',*,*,#3077,.F.);
#4119=ORIENTED_EDGE('',*,*,#2994,.T.);
#4120=ORIENTED_EDGE('',*,*,#3078,.F.);
#4121=ORIENTED_EDGE('',*,*,#3079,.F.);
#4122=ORIENTED_EDGE('',*,*,#3037,.T.);
#4123=ORIENTED_EDGE('',*,*,#3003,.T.);
#4124=ORIENTED_EDGE('',*,*,#3077,.T.);
#4125=ORIENTED_EDGE('',*,*,#3080,.F.);
#4126=ORIENTED_EDGE('',*,*,#3081,.T.);
#4127=ORIENTED_EDGE('',*,*,#2997,.T.);
#4128=ORIENTED_EDGE('',*,*,#3082,.T.);
#4129=ORIENTED_EDGE('',*,*,#3083,.T.);
#4130=ORIENTED_EDGE('',*,*,#3078,.T.);
#4131=ORIENTED_EDGE('',*,*,#3004,.T.);
#4132=ORIENTED_EDGE('',*,*,#3081,.F.);
#4133=ORIENTED_EDGE('',*,*,#3084,.F.);
#4134=ORIENTED_EDGE('',*,*,#3032,.F.);
#4135=ORIENTED_EDGE('',*,*,#2996,.T.);
#4136=ORIENTED_EDGE('',*,*,#3036,.F.);
#4137=ORIENTED_EDGE('',*,*,#3085,.F.);
#4138=ORIENTED_EDGE('',*,*,#3082,.F.);
#4139=ORIENTED_EDGE('',*,*,#3055,.T.);
#4140=ORIENTED_EDGE('',*,*,#3044,.T.);
#4141=ORIENTED_EDGE('',*,*,#3059,.T.);
#4142=ORIENTED_EDGE('',*,*,#3063,.F.);
#4143=ORIENTED_EDGE('',*,*,#3065,.T.);
#4144=ORIENTED_EDGE('',*,*,#3041,.T.);
#4145=ORIENTED_EDGE('',*,*,#3069,.T.);
#4146=ORIENTED_EDGE('',*,*,#3073,.F.);
#4147=ORIENTED_EDGE('',*,*,#3075,.T.);
#4148=ORIENTED_EDGE('',*,*,#3038,.T.);
#4149=ORIENTED_EDGE('',*,*,#3079,.T.);
#4150=ORIENTED_EDGE('',*,*,#3083,.F.);
#4151=ORIENTED_EDGE('',*,*,#3085,.T.);
#4152=ORIENTED_EDGE('',*,*,#3035,.T.);
#4153=ORIENTED_EDGE('',*,*,#3086,.T.);
#4154=ORIENTED_EDGE('',*,*,#3087,.T.);
#4155=ORIENTED_EDGE('',*,*,#3088,.F.);
#4156=ORIENTED_EDGE('',*,*,#3019,.T.);
#4157=ORIENTED_EDGE('',*,*,#3049,.T.);
#4158=ORIENTED_EDGE('',*,*,#3053,.F.);
#4159=ORIENTED_EDGE('',*,*,#3034,.T.);
#4160=ORIENTED_EDGE('',*,*,#3089,.F.);
#4161=ORIENTED_EDGE('',*,*,#3090,.F.);
#4162=ORIENTED_EDGE('',*,*,#3086,.F.);
#4163=ORIENTED_EDGE('',*,*,#3054,.T.);
#4164=ORIENTED_EDGE('',*,*,#3050,.T.);
#4165=ORIENTED_EDGE('',*,*,#3046,.T.);
#4166=ORIENTED_EDGE('',*,*,#3021,.T.);
#4167=ORIENTED_EDGE('',*,*,#3091,.F.);
#4168=ORIENTED_EDGE('',*,*,#3092,.F.);
#4169=ORIENTED_EDGE('',*,*,#3089,.T.);
#4170=ORIENTED_EDGE('',*,*,#3033,.T.);
#4171=ORIENTED_EDGE('',*,*,#3084,.T.);
#4172=ORIENTED_EDGE('',*,*,#3080,.T.);
#4173=ORIENTED_EDGE('',*,*,#3076,.T.);
#4174=ORIENTED_EDGE('',*,*,#3030,.T.);
#4175=ORIENTED_EDGE('',*,*,#3074,.T.);
#4176=ORIENTED_EDGE('',*,*,#3070,.T.);
#4177=ORIENTED_EDGE('',*,*,#3066,.T.);
#4178=ORIENTED_EDGE('',*,*,#3027,.T.);
#4179=ORIENTED_EDGE('',*,*,#3064,.T.);
#4180=ORIENTED_EDGE('',*,*,#3060,.T.);
#4181=ORIENTED_EDGE('',*,*,#3056,.T.);
#4182=ORIENTED_EDGE('',*,*,#3024,.T.);
#4183=ORIENTED_EDGE('',*,*,#3090,.T.);
#4184=ORIENTED_EDGE('',*,*,#3092,.T.);
#4185=ORIENTED_EDGE('',*,*,#3093,.F.);
#4186=ORIENTED_EDGE('',*,*,#3087,.F.);
#4187=ORIENTED_EDGE('',*,*,#2985,.T.);
#4188=ORIENTED_EDGE('',*,*,#2982,.T.);
#4189=ORIENTED_EDGE('',*,*,#2977,.T.);
#4190=ORIENTED_EDGE('',*,*,#2974,.T.);
#4191=ORIENTED_EDGE('',*,*,#2971,.T.);
#4192=ORIENTED_EDGE('',*,*,#2968,.T.);
#4193=ORIENTED_EDGE('',*,*,#3020,.T.);
#4194=ORIENTED_EDGE('',*,*,#3088,.T.);
#4195=ORIENTED_EDGE('',*,*,#3093,.T.);
#4196=ORIENTED_EDGE('',*,*,#3091,.T.);
#5308=PLANE('',#6012);
#5309=PLANE('',#6016);
#5310=PLANE('',#6020);
#5311=PLANE('',#6024);
#5312=PLANE('',#6031);
#5313=PLANE('',#6032);
#5314=PLANE('',#6033);
#5315=PLANE('',#6034);
#5316=PLANE('',#6035);
#5317=PLANE('',#6036);
#5318=PLANE('',#6037);
#5319=PLANE('',#6038);
#5320=PLANE('',#6039);
#5321=PLANE('',#6040);
#5322=PLANE('',#6041);
#5323=PLANE('',#6042);
#5324=PLANE('',#6043);
#5325=PLANE('',#6044);
#5326=PLANE('',#6045);
#5327=PLANE('',#6046);
#5328=PLANE('',#6047);
#5329=PLANE('',#6048);
#5330=PLANE('',#6049);
#5331=PLANE('',#6050);
#5332=PLANE('',#6051);
#5333=PLANE('',#6052);
#5334=PLANE('',#6053);
#5335=PLANE('',#6054);
#5336=PLANE('',#6055);
#5337=PLANE('',#6056);
#5338=PLANE('',#6057);
#5339=PLANE('',#6058);
#5340=PLANE('',#6059);
#5341=PLANE('',#6060);
#5342=PLANE('',#6061);
#5343=PLANE('',#6062);
#5344=PLANE('',#6063);
#5345=PLANE('',#6064);
#5346=PLANE('',#6065);
#5347=PLANE('',#6066);
#5348=PLANE('',#6067);
#5349=PLANE('',#6068);
#5511=ADVANCED_FACE('',(#697),#510,.F.);
#5512=ADVANCED_FACE('',(#698),#5308,.F.);
#5513=ADVANCED_FACE('',(#699),#511,.F.);
#5514=ADVANCED_FACE('',(#700),#5309,.F.);
#5515=ADVANCED_FACE('',(#701),#512,.F.);
#5516=ADVANCED_FACE('',(#702),#5310,.F.);
#5517=ADVANCED_FACE('',(#703),#513,.F.);
#5518=ADVANCED_FACE('',(#704),#5311,.F.);
#5519=ADVANCED_FACE('',(#705),#514,.F.);
#5520=ADVANCED_FACE('',(#706),#515,.F.);
#5521=ADVANCED_FACE('',(#707),#5312,.F.);
#5522=ADVANCED_FACE('',(#708),#5313,.F.);
#5523=ADVANCED_FACE('',(#709),#5314,.F.);
#5524=ADVANCED_FACE('',(#710),#5315,.F.);
#5525=ADVANCED_FACE('',(#711),#5316,.F.);
#5526=ADVANCED_FACE('',(#712),#5317,.F.);
#5527=ADVANCED_FACE('',(#713),#5318,.F.);
#5528=ADVANCED_FACE('',(#714),#5319,.F.);
#5529=ADVANCED_FACE('',(#715),#5320,.F.);
#5530=ADVANCED_FACE('',(#716),#5321,.T.);
#5531=ADVANCED_FACE('',(#717),#5322,.T.);
#5532=ADVANCED_FACE('',(#718),#5323,.T.);
#5533=ADVANCED_FACE('',(#719),#5324,.T.);
#5534=ADVANCED_FACE('',(#720),#5325,.F.);
#5535=ADVANCED_FACE('',(#721),#5326,.F.);
#5536=ADVANCED_FACE('',(#722),#5327,.T.);
#5537=ADVANCED_FACE('',(#723),#5328,.T.);
#5538=ADVANCED_FACE('',(#724,#401),#5329,.T.);
#5539=ADVANCED_FACE('',(#725),#5330,.T.);
#5540=ADVANCED_FACE('',(#726),#5331,.F.);
#5541=ADVANCED_FACE('',(#727),#5332,.F.);
#5542=ADVANCED_FACE('',(#728),#5333,.T.);
#5543=ADVANCED_FACE('',(#729),#5334,.T.);
#5544=ADVANCED_FACE('',(#730,#402),#5335,.T.);
#5545=ADVANCED_FACE('',(#731),#5336,.T.);
#5546=ADVANCED_FACE('',(#732),#5337,.F.);
#5547=ADVANCED_FACE('',(#733),#5338,.F.);
#5548=ADVANCED_FACE('',(#734),#5339,.T.);
#5549=ADVANCED_FACE('',(#735),#5340,.T.);
#5550=ADVANCED_FACE('',(#736),#5341,.T.);
#5551=ADVANCED_FACE('',(#737),#5342,.T.);
#5552=ADVANCED_FACE('',(#738),#5343,.F.);
#5553=ADVANCED_FACE('',(#739),#5344,.F.);
#5554=ADVANCED_FACE('',(#740),#5345,.T.);
#5555=ADVANCED_FACE('',(#741),#5346,.F.);
#5556=ADVANCED_FACE('',(#742),#5347,.T.);
#5557=ADVANCED_FACE('',(#743,#403,#404,#405,#406,#407,#408),#5348,.T.);
#5558=ADVANCED_FACE('',(#744),#5349,.T.);
#5721=CLOSED_SHELL('',(#5511,#5512,#5513,#5514,#5515,#5516,#5517,#5518,
#5519,#5520,#5521,#5522,#5523,#5524,#5525,#5526,#5527,#5528,#5529,#5530,
#5531,#5532,#5533,#5534,#5535,#5536,#5537,#5538,#5539,#5540,#5541,#5542,
#5543,#5544,#5545,#5546,#5547,#5548,#5549,#5550,#5551,#5552,#5553,#5554,
#5555,#5556,#5557,#5558));
#6008=AXIS2_PLACEMENT_3D('',#7898,#6625,#6626);
#6009=AXIS2_PLACEMENT_3D('',#7899,#6627,#6628);
#6010=AXIS2_PLACEMENT_3D('',#7901,#6629,#6630);
#6011=AXIS2_PLACEMENT_3D('',#7904,#6632,#6633);
#6012=AXIS2_PLACEMENT_3D('',#7905,#6634,#6635);
#6013=AXIS2_PLACEMENT_3D('',#7906,#6636,#6637);
#6014=AXIS2_PLACEMENT_3D('',#7908,#6638,#6639);
#6015=AXIS2_PLACEMENT_3D('',#7911,#6641,#6642);
#6016=AXIS2_PLACEMENT_3D('',#7912,#6643,#6644);
#6017=AXIS2_PLACEMENT_3D('',#7913,#6645,#6646);
#6018=AXIS2_PLACEMENT_3D('',#7915,#6647,#6648);
#6019=AXIS2_PLACEMENT_3D('',#7918,#6650,#6651);
#6020=AXIS2_PLACEMENT_3D('',#7919,#6652,#6653);
#6021=AXIS2_PLACEMENT_3D('',#7920,#6654,#6655);
#6022=AXIS2_PLACEMENT_3D('',#7922,#6656,#6657);
#6023=AXIS2_PLACEMENT_3D('',#7925,#6659,#6660);
#6024=AXIS2_PLACEMENT_3D('',#7926,#6661,#6662);
#6025=AXIS2_PLACEMENT_3D('',#7927,#6663,#6664);
#6026=AXIS2_PLACEMENT_3D('',#7929,#6665,#6666);
#6027=AXIS2_PLACEMENT_3D('',#7932,#6668,#6669);
#6028=AXIS2_PLACEMENT_3D('',#7933,#6670,#6671);
#6029=AXIS2_PLACEMENT_3D('',#7935,#6672,#6673);
#6030=AXIS2_PLACEMENT_3D('',#7938,#6675,#6676);
#6031=AXIS2_PLACEMENT_3D('',#7939,#6677,#6678);
#6032=AXIS2_PLACEMENT_3D('',#7948,#6683,#6684);
#6033=AXIS2_PLACEMENT_3D('',#7957,#6689,#6690);
#6034=AXIS2_PLACEMENT_3D('',#7966,#6695,#6696);
#6035=AXIS2_PLACEMENT_3D('',#7975,#6701,#6702);
#6036=AXIS2_PLACEMENT_3D('',#7984,#6707,#6708);
#6037=AXIS2_PLACEMENT_3D('',#7993,#6713,#6714);
#6038=AXIS2_PLACEMENT_3D('',#8002,#6719,#6720);
#6039=AXIS2_PLACEMENT_3D('',#8011,#6725,#6726);
#6040=AXIS2_PLACEMENT_3D('',#8060,#6755,#6756);
#6041=AXIS2_PLACEMENT_3D('',#8064,#6759,#6760);
#6042=AXIS2_PLACEMENT_3D('',#8068,#6763,#6764);
#6043=AXIS2_PLACEMENT_3D('',#8072,#6767,#6768);
#6044=AXIS2_PLACEMENT_3D('',#8076,#6771,#6772);
#6045=AXIS2_PLACEMENT_3D('',#8078,#6774,#6775);
#6046=AXIS2_PLACEMENT_3D('',#8080,#6777,#6778);
#6047=AXIS2_PLACEMENT_3D('',#8084,#6781,#6782);
#6048=AXIS2_PLACEMENT_3D('',#8088,#6785,#6786);
#6049=AXIS2_PLACEMENT_3D('',#8092,#6789,#6790);
#6050=AXIS2_PLACEMENT_3D('',#8096,#6793,#6794);
#6051=AXIS2_PLACEMENT_3D('',#8098,#6796,#6797);
#6052=AXIS2_PLACEMENT_3D('',#8100,#6799,#6800);
#6053=AXIS2_PLACEMENT_3D('',#8104,#6803,#6804);
#6054=AXIS2_PLACEMENT_3D('',#8108,#6807,#6808);
#6055=AXIS2_PLACEMENT_3D('',#8112,#6811,#6812);
#6056=AXIS2_PLACEMENT_3D('',#8116,#6815,#6816);
#6057=AXIS2_PLACEMENT_3D('',#8118,#6818,#6819);
#6058=AXIS2_PLACEMENT_3D('',#8120,#6821,#6822);
#6059=AXIS2_PLACEMENT_3D('',#8124,#6825,#6826);
#6060=AXIS2_PLACEMENT_3D('',#8128,#6829,#6830);
#6061=AXIS2_PLACEMENT_3D('',#8132,#6833,#6834);
#6062=AXIS2_PLACEMENT_3D('',#8136,#6837,#6838);
#6063=AXIS2_PLACEMENT_3D('',#8138,#6840,#6841);
#6064=AXIS2_PLACEMENT_3D('',#8140,#6843,#6844);
#6065=AXIS2_PLACEMENT_3D('',#8146,#6848,#6849);
#6066=AXIS2_PLACEMENT_3D('',#8150,#6852,#6853);
#6067=AXIS2_PLACEMENT_3D('',#8154,#6856,#6857);
#6068=AXIS2_PLACEMENT_3D('',#8156,#6859,#6860);
#6625=DIRECTION('axis',(0.,0.,1.));
#6626=DIRECTION('refdir',(1.,0.,0.));
#6627=DIRECTION('center_axis',(1.,0.,0.));
#6628=DIRECTION('ref_axis',(0.,0.,-1.));
#6629=DIRECTION('center_axis',(1.,0.,0.));
#6630=DIRECTION('ref_axis',(0.,0.,-1.));
#6631=DIRECTION('',(1.,0.,0.));
#6632=DIRECTION('center_axis',(1.,0.,0.));
#6633=DIRECTION('ref_axis',(0.,0.,-1.));
#6634=DIRECTION('center_axis',(1.,0.,0.));
#6635=DIRECTION('ref_axis',(0.,0.,-1.));
#6636=DIRECTION('center_axis',(1.,0.,0.));
#6637=DIRECTION('ref_axis',(0.,0.,-1.));
#6638=DIRECTION('center_axis',(1.,0.,0.));
#6639=DIRECTION('ref_axis',(0.,0.,-1.));
#6640=DIRECTION('',(1.,0.,0.));
#6641=DIRECTION('center_axis',(1.,0.,0.));
#6642=DIRECTION('ref_axis',(0.,0.,-1.));
#6643=DIRECTION('center_axis',(1.,0.,0.));
#6644=DIRECTION('ref_axis',(0.,0.,-1.));
#6645=DIRECTION('center_axis',(1.,0.,0.));
#6646=DIRECTION('ref_axis',(0.,0.,-1.));
#6647=DIRECTION('center_axis',(1.,0.,0.));
#6648=DIRECTION('ref_axis',(0.,0.,-1.));
#6649=DIRECTION('',(1.,0.,0.));
#6650=DIRECTION('center_axis',(1.,0.,0.));
#6651=DIRECTION('ref_axis',(0.,0.,-1.));
#6652=DIRECTION('center_axis',(1.,0.,0.));
#6653=DIRECTION('ref_axis',(0.,0.,-1.));
#6654=DIRECTION('center_axis',(1.,0.,0.));
#6655=DIRECTION('ref_axis',(0.,0.,-1.));
#6656=DIRECTION('center_axis',(1.,0.,0.));
#6657=DIRECTION('ref_axis',(0.,0.,-1.));
#6658=DIRECTION('',(1.,0.,0.));
#6659=DIRECTION('center_axis',(1.,0.,0.));
#6660=DIRECTION('ref_axis',(0.,0.,-1.));
#6661=DIRECTION('center_axis',(1.,0.,0.));
#6662=DIRECTION('ref_axis',(0.,0.,-1.));
#6663=DIRECTION('center_axis',(-1.,0.,0.));
#6664=DIRECTION('ref_axis',(0.,0.,-1.));
#6665=DIRECTION('center_axis',(-1.,0.,0.));
#6666=DIRECTION('ref_axis',(0.,0.,-1.));
#6667=DIRECTION('',(-1.,0.,0.));
#6668=DIRECTION('center_axis',(1.,0.,0.));
#6669=DIRECTION('ref_axis',(0.,0.,-1.));
#6670=DIRECTION('center_axis',(-1.,0.,0.));
#6671=DIRECTION('ref_axis',(0.,0.,-1.));
#6672=DIRECTION('center_axis',(-1.,0.,0.));
#6673=DIRECTION('ref_axis',(0.,0.,-1.));
#6674=DIRECTION('',(-1.,0.,0.));
#6675=DIRECTION('center_axis',(1.,0.,0.));
#6676=DIRECTION('ref_axis',(0.,0.,-1.));
#6677=DIRECTION('center_axis',(0.,1.,0.));
#6678=DIRECTION('ref_axis',(-1.,0.,0.));
#6679=DIRECTION('',(1.,0.,0.));
#6680=DIRECTION('',(0.,0.,1.));
#6681=DIRECTION('',(-1.,0.,0.));
#6682=DIRECTION('',(0.,0.,-1.));
#6683=DIRECTION('center_axis',(0.,1.,0.));
#6684=DIRECTION('ref_axis',(-1.,0.,0.));
#6685=DIRECTION('',(1.,0.,0.));
#6686=DIRECTION('',(0.,0.,1.));
#6687=DIRECTION('',(-1.,0.,0.));
#6688=DIRECTION('',(0.,0.,-1.));
#6689=DIRECTION('center_axis',(0.,1.,0.));
#6690=DIRECTION('ref_axis',(-1.,0.,0.));
#6691=DIRECTION('',(1.,0.,0.));
#6692=DIRECTION('',(0.,0.,1.));
#6693=DIRECTION('',(-1.,0.,0.));
#6694=DIRECTION('',(0.,0.,-1.));
#6695=DIRECTION('center_axis',(0.,1.,0.));
#6696=DIRECTION('ref_axis',(-1.,0.,0.));
#6697=DIRECTION('',(1.,0.,0.));
#6698=DIRECTION('',(0.,0.,1.));
#6699=DIRECTION('',(-1.,0.,0.));
#6700=DIRECTION('',(0.,0.,-1.));
#6701=DIRECTION('center_axis',(0.,-1.,0.));
#6702=DIRECTION('ref_axis',(1.,0.,0.));
#6703=DIRECTION('',(-1.,0.,0.));
#6704=DIRECTION('',(0.,0.,1.));
#6705=DIRECTION('',(1.,0.,0.));
#6706=DIRECTION('',(0.,0.,1.));
#6707=DIRECTION('center_axis',(0.,-1.,0.));
#6708=DIRECTION('ref_axis',(1.,0.,0.));
#6709=DIRECTION('',(-1.,0.,0.));
#6710=DIRECTION('',(0.,0.,1.));
#6711=DIRECTION('',(1.,0.,0.));
#6712=DIRECTION('',(0.,0.,1.));
#6713=DIRECTION('center_axis',(0.,-1.,0.));
#6714=DIRECTION('ref_axis',(1.,0.,0.));
#6715=DIRECTION('',(-1.,0.,0.));
#6716=DIRECTION('',(0.,0.,1.));
#6717=DIRECTION('',(1.,0.,0.));
#6718=DIRECTION('',(0.,0.,1.));
#6719=DIRECTION('center_axis',(0.,-1.,0.));
#6720=DIRECTION('ref_axis',(1.,0.,0.));
#6721=DIRECTION('',(-1.,0.,0.));
#6722=DIRECTION('',(0.,0.,1.));
#6723=DIRECTION('',(1.,0.,0.));
#6724=DIRECTION('',(0.,0.,1.));
#6725=DIRECTION('center_axis',(-1.,0.,0.));
#6726=DIRECTION('ref_axis',(0.,-1.,0.));
#6727=DIRECTION('',(0.,-1.,0.));
#6728=DIRECTION('',(0.,0.,-1.));
#6729=DIRECTION('',(0.,1.,0.));
#6730=DIRECTION('',(0.,0.,1.));
#6731=DIRECTION('',(0.,-1.,0.));
#6732=DIRECTION('',(0.,-1.,0.));
#6733=DIRECTION('',(0.,0.,1.));
#6734=DIRECTION('',(0.,-1.,0.));
#6735=DIRECTION('',(0.,-1.,0.));
#6736=DIRECTION('',(0.,0.,1.));
#6737=DIRECTION('',(0.,-1.,0.));
#6738=DIRECTION('',(0.,-1.,0.));
#6739=DIRECTION('',(0.,0.,1.));
#6740=DIRECTION('',(0.,-1.,0.));
#6741=DIRECTION('',(0.,-1.,0.));
#6742=DIRECTION('',(0.,0.,1.));
#6743=DIRECTION('',(0.,-1.,0.));
#6744=DIRECTION('',(0.,0.,-1.));
#6745=DIRECTION('',(0.,-1.,0.));
#6746=DIRECTION('',(0.,-1.,0.));
#6747=DIRECTION('',(0.,0.,-1.));
#6748=DIRECTION('',(0.,-1.,0.));
#6749=DIRECTION('',(0.,-1.,0.));
#6750=DIRECTION('',(0.,0.,-1.));
#6751=DIRECTION('',(0.,-1.,0.));
#6752=DIRECTION('',(0.,-1.,0.));
#6753=DIRECTION('',(0.,0.,-1.));
#6754=DIRECTION('',(0.,-1.,0.));
#6755=DIRECTION('center_axis',(0.,0.,1.));
#6756=DIRECTION('ref_axis',(1.,0.,0.));
#6757=DIRECTION('',(-1.,0.,0.));
#6758=DIRECTION('',(0.,-1.,0.));
#6759=DIRECTION('center_axis',(0.,0.,1.));
#6760=DIRECTION('ref_axis',(1.,0.,0.));
#6761=DIRECTION('',(0.,-1.,0.));
#6762=DIRECTION('',(1.,0.,0.));
#6763=DIRECTION('center_axis',(1.,0.,0.));
#6764=DIRECTION('ref_axis',(0.,1.,0.));
#6765=DIRECTION('',(0.,0.,1.));
#6766=DIRECTION('',(0.,1.,0.));
#6767=DIRECTION('center_axis',(1.,0.,0.));
#6768=DIRECTION('ref_axis',(0.,1.,0.));
#6769=DIRECTION('',(0.,1.,0.));
#6770=DIRECTION('',(0.,0.,1.));
#6771=DIRECTION('center_axis',(0.,0.,1.));
#6772=DIRECTION('ref_axis',(1.,0.,0.));
#6773=DIRECTION('',(1.,0.,0.));
#6774=DIRECTION('center_axis',(0.,0.,1.));
#6775=DIRECTION('ref_axis',(1.,0.,0.));
#6776=DIRECTION('',(-1.,0.,0.));
#6777=DIRECTION('center_axis',(0.,0.,1.));
#6778=DIRECTION('ref_axis',(1.,0.,0.));
#6779=DIRECTION('',(-1.,0.,0.));
#6780=DIRECTION('',(0.,-1.,0.));
#6781=DIRECTION('center_axis',(0.,0.,1.));
#6782=DIRECTION('ref_axis',(1.,0.,0.));
#6783=DIRECTION('',(0.,-1.,0.));
#6784=DIRECTION('',(1.,0.,0.));
#6785=DIRECTION('center_axis',(1.,0.,0.));
#6786=DIRECTION('ref_axis',(0.,1.,0.));
#6787=DIRECTION('',(0.,0.,1.));
#6788=DIRECTION('',(0.,1.,0.));
#6789=DIRECTION('center_axis',(1.,0.,0.));
#6790=DIRECTION('ref_axis',(0.,1.,0.));
#6791=DIRECTION('',(0.,1.,0.));
#6792=DIRECTION('',(0.,0.,1.));
#6793=DIRECTION('center_axis',(0.,0.,1.));
#6794=DIRECTION('ref_axis',(1.,0.,0.));
#6795=DIRECTION('',(1.,0.,0.));
#6796=DIRECTION('center_axis',(0.,0.,1.));
#6797=DIRECTION('ref_axis',(1.,0.,0.));
#6798=DIRECTION('',(-1.,0.,0.));
#6799=DIRECTION('center_axis',(0.,0.,1.));
#6800=DIRECTION('ref_axis',(1.,0.,0.));
#6801=DIRECTION('',(-1.,0.,0.));
#6802=DIRECTION('',(0.,-1.,0.));
#6803=DIRECTION('center_axis',(0.,0.,1.));
#6804=DIRECTION('ref_axis',(1.,0.,0.));
#6805=DIRECTION('',(0.,-1.,0.));
#6806=DIRECTION('',(1.,0.,0.));
#6807=DIRECTION('center_axis',(1.,0.,0.));
#6808=DIRECTION('ref_axis',(0.,1.,0.));
#6809=DIRECTION('',(0.,0.,1.));
#6810=DIRECTION('',(0.,1.,0.));
#6811=DIRECTION('center_axis',(1.,0.,0.));
#6812=DIRECTION('ref_axis',(0.,1.,0.));
#6813=DIRECTION('',(0.,1.,0.));
#6814=DIRECTION('',(0.,0.,1.));
#6815=DIRECTION('center_axis',(0.,0.,1.));
#6816=DIRECTION('ref_axis',(1.,0.,0.));
#6817=DIRECTION('',(1.,0.,0.));
#6818=DIRECTION('center_axis',(0.,0.,1.));
#6819=DIRECTION('ref_axis',(1.,0.,0.));
#6820=DIRECTION('',(-1.,0.,0.));
#6821=DIRECTION('center_axis',(0.,0.,1.));
#6822=DIRECTION('ref_axis',(1.,0.,0.));
#6823=DIRECTION('',(-1.,0.,0.));
#6824=DIRECTION('',(0.,-1.,0.));
#6825=DIRECTION('center_axis',(0.,0.,1.));
#6826=DIRECTION('ref_axis',(1.,0.,0.));
#6827=DIRECTION('',(0.,-1.,0.));
#6828=DIRECTION('',(1.,0.,0.));
#6829=DIRECTION('center_axis',(1.,0.,0.));
#6830=DIRECTION('ref_axis',(0.,1.,0.));
#6831=DIRECTION('',(0.,0.,1.));
#6832=DIRECTION('',(0.,1.,0.));
#6833=DIRECTION('center_axis',(1.,0.,0.));
#6834=DIRECTION('ref_axis',(0.,1.,0.));
#6835=DIRECTION('',(0.,1.,0.));
#6836=DIRECTION('',(0.,0.,1.));
#6837=DIRECTION('center_axis',(0.,0.,1.));
#6838=DIRECTION('ref_axis',(1.,0.,0.));
#6839=DIRECTION('',(1.,0.,0.));
#6840=DIRECTION('center_axis',(0.,0.,1.));
#6841=DIRECTION('ref_axis',(1.,0.,0.));
#6842=DIRECTION('',(-1.,0.,0.));
#6843=DIRECTION('center_axis',(0.,1.,0.));
#6844=DIRECTION('ref_axis',(-1.,0.,0.));
#6845=DIRECTION('',(-1.,0.,0.));
#6846=DIRECTION('',(0.,0.,1.));
#6847=DIRECTION('',(-1.,0.,0.));
#6848=DIRECTION('center_axis',(0.,0.,1.));
#6849=DIRECTION('ref_axis',(1.,0.,0.));
#6850=DIRECTION('',(1.,0.,0.));
#6851=DIRECTION('',(0.,-1.,0.));
#6852=DIRECTION('center_axis',(0.,-1.,0.));
#6853=DIRECTION('ref_axis',(1.,0.,0.));
#6854=DIRECTION('',(1.,0.,0.));
#6855=DIRECTION('',(0.,0.,1.));
#6856=DIRECTION('center_axis',(-1.,0.,0.));
#6857=DIRECTION('ref_axis',(0.,-1.,0.));
#6858=DIRECTION('',(0.,-1.,0.));
#6859=DIRECTION('center_axis',(0.,0.,1.));
#6860=DIRECTION('ref_axis',(1.,0.,0.));
#7898=CARTESIAN_POINT('',(0.,0.,0.));
#7899=CARTESIAN_POINT('Origin',(0.,51.,60.));
#7900=CARTESIAN_POINT('',(0.,51.,60.41));
#7901=CARTESIAN_POINT('Origin',(0.,51.,60.));
#7902=CARTESIAN_POINT('',(1.5,51.,60.41));
#7903=CARTESIAN_POINT('',(0.,51.,60.41));
#7904=CARTESIAN_POINT('Origin',(1.5,51.,60.));
#7905=CARTESIAN_POINT('Origin',(1.5,51.,60.));
#7906=CARTESIAN_POINT('Origin',(0.,9.,120.));
#7907=CARTESIAN_POINT('',(0.,9.,120.41));
#7908=CARTESIAN_POINT('Origin',(0.,9.,120.));
#7909=CARTESIAN_POINT('',(1.5,9.,120.41));
#7910=CARTESIAN_POINT('',(0.,9.,120.41));
#7911=CARTESIAN_POINT('Origin',(1.5,9.,120.));
#7912=CARTESIAN_POINT('Origin',(1.5,9.,120.));
#7913=CARTESIAN_POINT('Origin',(0.,9.,60.));
#7914=CARTESIAN_POINT('',(0.,9.,60.41));
#7915=CARTESIAN_POINT('Origin',(0.,9.,60.));
#7916=CARTESIAN_POINT('',(1.5,9.,60.41));
#7917=CARTESIAN_POINT('',(0.,9.,60.41));
#7918=CARTESIAN_POINT('Origin',(1.5,9.,60.));
#7919=CARTESIAN_POINT('Origin',(1.5,9.,60.));
#7920=CARTESIAN_POINT('Origin',(0.,51.,120.));
#7921=CARTESIAN_POINT('',(0.,51.,120.41));
#7922=CARTESIAN_POINT('Origin',(0.,51.,120.));
#7923=CARTESIAN_POINT('',(1.5,51.,120.41));
#7924=CARTESIAN_POINT('',(0.,51.,120.41));
#7925=CARTESIAN_POINT('Origin',(1.5,51.,120.));
#7926=CARTESIAN_POINT('Origin',(1.5,51.,120.));
#7927=CARTESIAN_POINT('Origin',(1.8,1.6,60.));
#7928=CARTESIAN_POINT('',(1.8,1.6,60.225));
#7929=CARTESIAN_POINT('Origin',(1.8,1.6,60.));
#7930=CARTESIAN_POINT('',(0.,1.6,60.225));
#7931=CARTESIAN_POINT('',(1.8,1.6,60.225));
#7932=CARTESIAN_POINT('Origin',(0.,1.6,60.));
#7933=CARTESIAN_POINT('Origin',(1.8,1.6,120.));
#7934=CARTESIAN_POINT('',(1.8,1.6,120.225));
#7935=CARTESIAN_POINT('Origin',(1.8,1.6,120.));
#7936=CARTESIAN_POINT('',(0.,1.6,120.225));
#7937=CARTESIAN_POINT('',(1.8,1.6,120.225));
#7938=CARTESIAN_POINT('Origin',(0.,1.6,120.));
#7939=CARTESIAN_POINT('Origin',(1.81,58.82,0.));
#7940=CARTESIAN_POINT('',(1.3,58.82,134.08));
#7941=CARTESIAN_POINT('',(1.8,58.82,134.08));
#7942=CARTESIAN_POINT('',(1.6825,58.82,134.08));
#7943=CARTESIAN_POINT('',(1.3,58.82,90.92));
#7944=CARTESIAN_POINT('',(1.3,58.82,0.));
#7945=CARTESIAN_POINT('',(1.8,58.82,90.92));
#7946=CARTESIAN_POINT('',(1.6825,58.82,90.92));
#7947=CARTESIAN_POINT('',(1.8,58.82,0.));
#7948=CARTESIAN_POINT('Origin',(1.81,58.82,0.));
#7949=CARTESIAN_POINT('',(1.3,58.82,89.08));
#7950=CARTESIAN_POINT('',(1.8,58.82,89.08));
#7951=CARTESIAN_POINT('',(1.6825,58.82,89.08));
#7952=CARTESIAN_POINT('',(1.3,58.82,45.92));
#7953=CARTESIAN_POINT('',(1.3,58.82,0.));
#7954=CARTESIAN_POINT('',(1.8,58.82,45.92));
#7955=CARTESIAN_POINT('',(1.6825,58.82,45.92));
#7956=CARTESIAN_POINT('',(1.8,58.82,0.));
#7957=CARTESIAN_POINT('Origin',(1.81,58.82,0.));
#7958=CARTESIAN_POINT('',(1.3,58.82,44.08));
#7959=CARTESIAN_POINT('',(1.8,58.82,44.08));
#7960=CARTESIAN_POINT('',(1.6825,58.82,44.08));
#7961=CARTESIAN_POINT('',(1.3,58.82,1.82));
#7962=CARTESIAN_POINT('',(1.3,58.82,0.));
#7963=CARTESIAN_POINT('',(1.8,58.82,1.82));
#7964=CARTESIAN_POINT('',(1.6825,58.82,1.82));
#7965=CARTESIAN_POINT('',(1.8,58.82,0.));
#7966=CARTESIAN_POINT('Origin',(1.81,58.82,0.));
#7967=CARTESIAN_POINT('',(1.3,58.82,178.18));
#7968=CARTESIAN_POINT('',(1.8,58.82,178.18));
#7969=CARTESIAN_POINT('',(1.6825,58.82,178.18));
#7970=CARTESIAN_POINT('',(1.3,58.82,135.92));
#7971=CARTESIAN_POINT('',(1.3,58.82,0.));
#7972=CARTESIAN_POINT('',(1.8,58.82,135.92));
#7973=CARTESIAN_POINT('',(1.6825,58.82,135.92));
#7974=CARTESIAN_POINT('',(1.8,58.82,0.));
#7975=CARTESIAN_POINT('Origin',(1.3,58.18,0.));
#7976=CARTESIAN_POINT('',(1.8,58.18,44.08));
#7977=CARTESIAN_POINT('',(1.3,58.18,44.08));
#7978=CARTESIAN_POINT('',(1.4275,58.18,44.08));
#7979=CARTESIAN_POINT('',(1.8,58.18,1.82));
#7980=CARTESIAN_POINT('',(1.8,58.18,0.));
#7981=CARTESIAN_POINT('',(1.3,58.18,1.82));
#7982=CARTESIAN_POINT('',(1.4275,58.18,1.82));
#7983=CARTESIAN_POINT('',(1.3,58.18,0.));
#7984=CARTESIAN_POINT('Origin',(1.3,58.18,0.));
#7985=CARTESIAN_POINT('',(1.8,58.18,89.08));
#7986=CARTESIAN_POINT('',(1.3,58.18,89.08));
#7987=CARTESIAN_POINT('',(1.4275,58.18,89.08));
#7988=CARTESIAN_POINT('',(1.8,58.18,45.92));
#7989=CARTESIAN_POINT('',(1.8,58.18,0.));
#7990=CARTESIAN_POINT('',(1.3,58.18,45.92));
#7991=CARTESIAN_POINT('',(1.4275,58.18,45.92));
#7992=CARTESIAN_POINT('',(1.3,58.18,0.));
#7993=CARTESIAN_POINT('Origin',(1.3,58.18,0.));
#7994=CARTESIAN_POINT('',(1.8,58.18,134.08));
#7995=CARTESIAN_POINT('',(1.3,58.18,134.08));
#7996=CARTESIAN_POINT('',(1.4275,58.18,134.08));
#7997=CARTESIAN_POINT('',(1.8,58.18,90.92));
#7998=CARTESIAN_POINT('',(1.8,58.18,0.));
#7999=CARTESIAN_POINT('',(1.3,58.18,90.92));
#8000=CARTESIAN_POINT('',(1.4275,58.18,90.92));
#8001=CARTESIAN_POINT('',(1.3,58.18,0.));
#8002=CARTESIAN_POINT('Origin',(1.3,58.18,0.));
#8003=CARTESIAN_POINT('',(1.8,58.18,178.18));
#8004=CARTESIAN_POINT('',(1.3,58.18,178.18));
#8005=CARTESIAN_POINT('',(1.4275,58.18,178.18));
#8006=CARTESIAN_POINT('',(1.8,58.18,135.92));
#8007=CARTESIAN_POINT('',(1.8,58.18,0.));
#8008=CARTESIAN_POINT('',(1.3,58.18,135.92));
#8009=CARTESIAN_POINT('',(1.4275,58.18,135.92));
#8010=CARTESIAN_POINT('',(1.3,58.18,0.));
#8011=CARTESIAN_POINT('Origin',(1.3,60.,178.18));
#8012=CARTESIAN_POINT('',(1.3,60.,178.18));
#8013=CARTESIAN_POINT('',(1.3,60.,178.18));
#8014=CARTESIAN_POINT('',(1.3,60.,180.));
#8015=CARTESIAN_POINT('',(1.3,60.,89.09));
#8016=CARTESIAN_POINT('',(1.3,0.,180.));
#8017=CARTESIAN_POINT('',(1.3,45.,180.));
#8018=CARTESIAN_POINT('',(1.3,0.,178.18));
#8019=CARTESIAN_POINT('',(1.3,0.,89.09));
#8020=CARTESIAN_POINT('',(1.3,60.,178.18));
#8021=CARTESIAN_POINT('',(1.3,0.,135.92));
#8022=CARTESIAN_POINT('',(1.3,60.,135.92));
#8023=CARTESIAN_POINT('',(1.3,0.,134.08));
#8024=CARTESIAN_POINT('',(1.3,0.,67.04));
#8025=CARTESIAN_POINT('',(1.3,60.,134.08));
#8026=CARTESIAN_POINT('',(1.3,0.,90.92));
#8027=CARTESIAN_POINT('',(1.3,60.,90.92));
#8028=CARTESIAN_POINT('',(1.3,0.,89.08));
#8029=CARTESIAN_POINT('',(1.3,0.,44.54));
#8030=CARTESIAN_POINT('',(1.3,60.,89.08));
#8031=CARTESIAN_POINT('',(1.3,0.,45.92));
#8032=CARTESIAN_POINT('',(1.3,60.,45.92));
#8033=CARTESIAN_POINT('',(1.3,0.,44.08));
#8034=CARTESIAN_POINT('',(1.3,0.,22.04));
#8035=CARTESIAN_POINT('',(1.3,60.,44.08));
#8036=CARTESIAN_POINT('',(1.3,0.,1.82));
#8037=CARTESIAN_POINT('',(1.3,60.,1.82));
#8038=CARTESIAN_POINT('',(1.3,0.,0.));
#8039=CARTESIAN_POINT('',(1.3,0.,0.));
#8040=CARTESIAN_POINT('',(1.3,60.,0.));
#8041=CARTESIAN_POINT('',(1.3,45.,0.));
#8042=CARTESIAN_POINT('',(1.3,60.,1.82));
#8043=CARTESIAN_POINT('',(1.3,60.,0.));
#8044=CARTESIAN_POINT('',(1.3,60.,1.82));
#8045=CARTESIAN_POINT('',(1.3,60.,44.08));
#8046=CARTESIAN_POINT('',(1.3,60.,44.08));
#8047=CARTESIAN_POINT('',(1.3,60.,45.92));
#8048=CARTESIAN_POINT('',(1.3,60.,22.04));
#8049=CARTESIAN_POINT('',(1.3,60.,45.92));
#8050=CARTESIAN_POINT('',(1.3,60.,89.08));
#8051=CARTESIAN_POINT('',(1.3,60.,89.08));
#8052=CARTESIAN_POINT('',(1.3,60.,90.92));
#8053=CARTESIAN_POINT('',(1.3,60.,44.54));
#8054=CARTESIAN_POINT('',(1.3,60.,90.92));
#8055=CARTESIAN_POINT('',(1.3,60.,134.08));
#8056=CARTESIAN_POINT('',(1.3,60.,134.08));
#8057=CARTESIAN_POINT('',(1.3,60.,135.92));
#8058=CARTESIAN_POINT('',(1.3,60.,67.04));
#8059=CARTESIAN_POINT('',(1.3,60.,135.92));
#8060=CARTESIAN_POINT('Origin',(1.555,30.,178.18));
#8061=CARTESIAN_POINT('',(1.8,0.,178.18));
#8062=CARTESIAN_POINT('',(0.7775,0.,178.18));
#8063=CARTESIAN_POINT('',(1.8,15.,178.18));
#8064=CARTESIAN_POINT('Origin',(1.555,30.,178.18));
#8065=CARTESIAN_POINT('',(1.8,60.,178.18));
#8066=CARTESIAN_POINT('',(1.8,15.,178.18));
#8067=CARTESIAN_POINT('',(1.6775,60.,178.18));
#8068=CARTESIAN_POINT('Origin',(1.8,0.,0.));
#8069=CARTESIAN_POINT('',(1.8,0.,135.92));
#8070=CARTESIAN_POINT('',(1.8,0.,0.));
#8071=CARTESIAN_POINT('',(1.8,15.,135.92));
#8072=CARTESIAN_POINT('Origin',(1.8,0.,0.));
#8073=CARTESIAN_POINT('',(1.8,60.,135.92));
#8074=CARTESIAN_POINT('',(1.8,15.,135.92));
#8075=CARTESIAN_POINT('',(1.8,60.,0.));
#8076=CARTESIAN_POINT('Origin',(1.555,30.,135.92));
#8077=CARTESIAN_POINT('',(0.7775,0.,135.92));
#8078=CARTESIAN_POINT('Origin',(1.555,30.,135.92));
#8079=CARTESIAN_POINT('',(1.6775,60.,135.92));
#8080=CARTESIAN_POINT('Origin',(1.555,30.,134.08));
#8081=CARTESIAN_POINT('',(1.8,0.,134.08));
#8082=CARTESIAN_POINT('',(0.7775,0.,134.08));
#8083=CARTESIAN_POINT('',(1.8,15.,134.08));
#8084=CARTESIAN_POINT('Origin',(1.555,30.,134.08));
#8085=CARTESIAN_POINT('',(1.8,60.,134.08));
#8086=CARTESIAN_POINT('',(1.8,15.,134.08));
#8087=CARTESIAN_POINT('',(1.6775,60.,134.08));
#8088=CARTESIAN_POINT('Origin',(1.8,0.,0.));
#8089=CARTESIAN_POINT('',(1.8,0.,90.92));
#8090=CARTESIAN_POINT('',(1.8,0.,0.));
#8091=CARTESIAN_POINT('',(1.8,15.,90.92));
#8092=CARTESIAN_POINT('Origin',(1.8,0.,0.));
#8093=CARTESIAN_POINT('',(1.8,60.,90.92));
#8094=CARTESIAN_POINT('',(1.8,15.,90.92));
#8095=CARTESIAN_POINT('',(1.8,60.,0.));
#8096=CARTESIAN_POINT('Origin',(1.555,30.,90.92));
#8097=CARTESIAN_POINT('',(0.7775,0.,90.92));
#8098=CARTESIAN_POINT('Origin',(1.555,30.,90.92));
#8099=CARTESIAN_POINT('',(1.6775,60.,90.92));
#8100=CARTESIAN_POINT('Origin',(1.555,30.,89.08));
#8101=CARTESIAN_POINT('',(1.8,0.,89.08));
#8102=CARTESIAN_POINT('',(0.7775,0.,89.08));
#8103=CARTESIAN_POINT('',(1.8,15.,89.08));
#8104=CARTESIAN_POINT('Origin',(1.555,30.,89.08));
#8105=CARTESIAN_POINT('',(1.8,60.,89.08));
#8106=CARTESIAN_POINT('',(1.8,15.,89.08));
#8107=CARTESIAN_POINT('',(1.6775,60.,89.08));
#8108=CARTESIAN_POINT('Origin',(1.8,0.,0.));
#8109=CARTESIAN_POINT('',(1.8,0.,45.92));
#8110=CARTESIAN_POINT('',(1.8,0.,0.));
#8111=CARTESIAN_POINT('',(1.8,15.,45.92));
#8112=CARTESIAN_POINT('Origin',(1.8,0.,0.));
#8113=CARTESIAN_POINT('',(1.8,60.,45.92));
#8114=CARTESIAN_POINT('',(1.8,15.,45.92));
#8115=CARTESIAN_POINT('',(1.8,60.,0.));
#8116=CARTESIAN_POINT('Origin',(1.555,30.,45.92));
#8117=CARTESIAN_POINT('',(0.7775,0.,45.92));
#8118=CARTESIAN_POINT('Origin',(1.555,30.,45.92));
#8119=CARTESIAN_POINT('',(1.6775,60.,45.92));
#8120=CARTESIAN_POINT('Origin',(1.555,30.,44.08));
#8121=CARTESIAN_POINT('',(1.8,0.,44.08));
#8122=CARTESIAN_POINT('',(0.7775,0.,44.08));
#8123=CARTESIAN_POINT('',(1.8,15.,44.08));
#8124=CARTESIAN_POINT('Origin',(1.555,30.,44.08));
#8125=CARTESIAN_POINT('',(1.8,60.,44.08));
#8126=CARTESIAN_POINT('',(1.8,15.,44.08));
#8127=CARTESIAN_POINT('',(1.6775,60.,44.08));
#8128=CARTESIAN_POINT('Origin',(1.8,0.,0.));
#8129=CARTESIAN_POINT('',(1.8,0.,1.82));
#8130=CARTESIAN_POINT('',(1.8,0.,0.));
#8131=CARTESIAN_POINT('',(1.8,15.,1.82));
#8132=CARTESIAN_POINT('Origin',(1.8,0.,0.));
#8133=CARTESIAN_POINT('',(1.8,60.,1.82));
#8134=CARTESIAN_POINT('',(1.8,15.,1.82));
#8135=CARTESIAN_POINT('',(1.8,60.,0.));
#8136=CARTESIAN_POINT('Origin',(1.555,30.,1.82));
#8137=CARTESIAN_POINT('',(0.7775,0.,1.82));
#8138=CARTESIAN_POINT('Origin',(1.555,30.,1.82));
#8139=CARTESIAN_POINT('',(1.6775,60.,1.82));
#8140=CARTESIAN_POINT('Origin',(1.8,60.,0.));
#8141=CARTESIAN_POINT('',(0.,60.,0.));
#8142=CARTESIAN_POINT('',(1.8,60.,0.));
#8143=CARTESIAN_POINT('',(0.,60.,180.));
#8144=CARTESIAN_POINT('',(0.,60.,0.));
#8145=CARTESIAN_POINT('',(1.8,60.,180.));
#8146=CARTESIAN_POINT('Origin',(0.9,30.,0.));
#8147=CARTESIAN_POINT('',(0.,0.,0.));
#8148=CARTESIAN_POINT('',(0.,0.,0.));
#8149=CARTESIAN_POINT('',(0.,60.,0.));
#8150=CARTESIAN_POINT('Origin',(0.,0.,0.));
#8151=CARTESIAN_POINT('',(0.,0.,180.));
#8152=CARTESIAN_POINT('',(0.,0.,180.));
#8153=CARTESIAN_POINT('',(0.,0.,0.));
#8154=CARTESIAN_POINT('Origin',(0.,60.,0.));
#8155=CARTESIAN_POINT('',(0.,60.,180.));
#8156=CARTESIAN_POINT('Origin',(0.9,30.,180.));
#31540=UNCERTAINTY_MEASURE_WITH_UNIT(LENGTH_MEASURE(0.001),#31567,
'DISTANCE_ACCURACY_VALUE',
'Maximum model space distance between geometric entities at asserted c
onnectivities');
#31549=UNCERTAINTY_MEASURE_WITH_UNIT(LENGTH_MEASURE(0.001),#31567,
'DISTANCE_ACCURACY_VALUE',
'Maximum model space distance between geometric entities at asserted c
onnectivities');
#31557=(
GEOMETRIC_REPRESENTATION_CONTEXT(3)
GLOBAL_UNCERTAINTY_ASSIGNED_CONTEXT((#31540))
GLOBAL_UNIT_ASSIGNED_CONTEXT((#31567,#31569,#31570))
REPRESENTATION_CONTEXT('','3D')
);
#31566=(
GEOMETRIC_REPRESENTATION_CONTEXT(3)
GLOBAL_UNCERTAINTY_ASSIGNED_CONTEXT((#31549))
GLOBAL_UNIT_ASSIGNED_CONTEXT((#31567,#31569,#31570))
REPRESENTATION_CONTEXT('','3D')
);
#31567=(
LENGTH_UNIT()
NAMED_UNIT(*)
SI_UNIT(.CENTI.,.METRE.)
);
#31569=(
NAMED_UNIT(*)
PLANE_ANGLE_UNIT()
SI_UNIT($,.RADIAN.)
);
#31570=(
NAMED_UNIT(*)
SI_UNIT($,.STERADIAN.)
SOLID_ANGLE_UNIT()
);
#31578=SHAPE_DEFINITION_REPRESENTATION(#31594,#31642);
#31594=PRODUCT_DEFINITION_SHAPE('',$,#31659);
#31642=SHAPE_REPRESENTATION('',(#6008),#31557);
#31651=PRODUCT_DEFINITION_CONTEXT('part definition',#31701,'design');
#31659=PRODUCT_DEFINITION('Universal side panel','Universal side panel',
#31675,#31651);
#31675=PRODUCT_DEFINITION_FORMATION('',$,#31710);
#31701=APPLICATION_CONTEXT(
'Core Data for Automotive Mechanical Design Process');
#31702=PRODUCT_CONTEXT('part definition',#31701,'mechanical');
#31710=PRODUCT('Universal side panel','Universal side panel',$,(#31702));
#31723=PRESENTATION_STYLE_ASSIGNMENT((#31730));
#31730=SURFACE_STYLE_USAGE(.BOTH.,#31737);
#31737=SURFACE_SIDE_STYLE('',(#31744));
#31744=SURFACE_STYLE_FILL_AREA(#31751);
#31751=FILL_AREA_STYLE('Opaque(24,59,110)',(#31758));
#31758=FILL_AREA_STYLE_COLOUR('Opaque(24,59,110)',#31765);
#31765=COLOUR_RGB('Opaque(24,59,110)',0.0941176470588235,0.231372549019608,
0.431372549019608);
ENDSEC;
END-ISO-10303-21;
